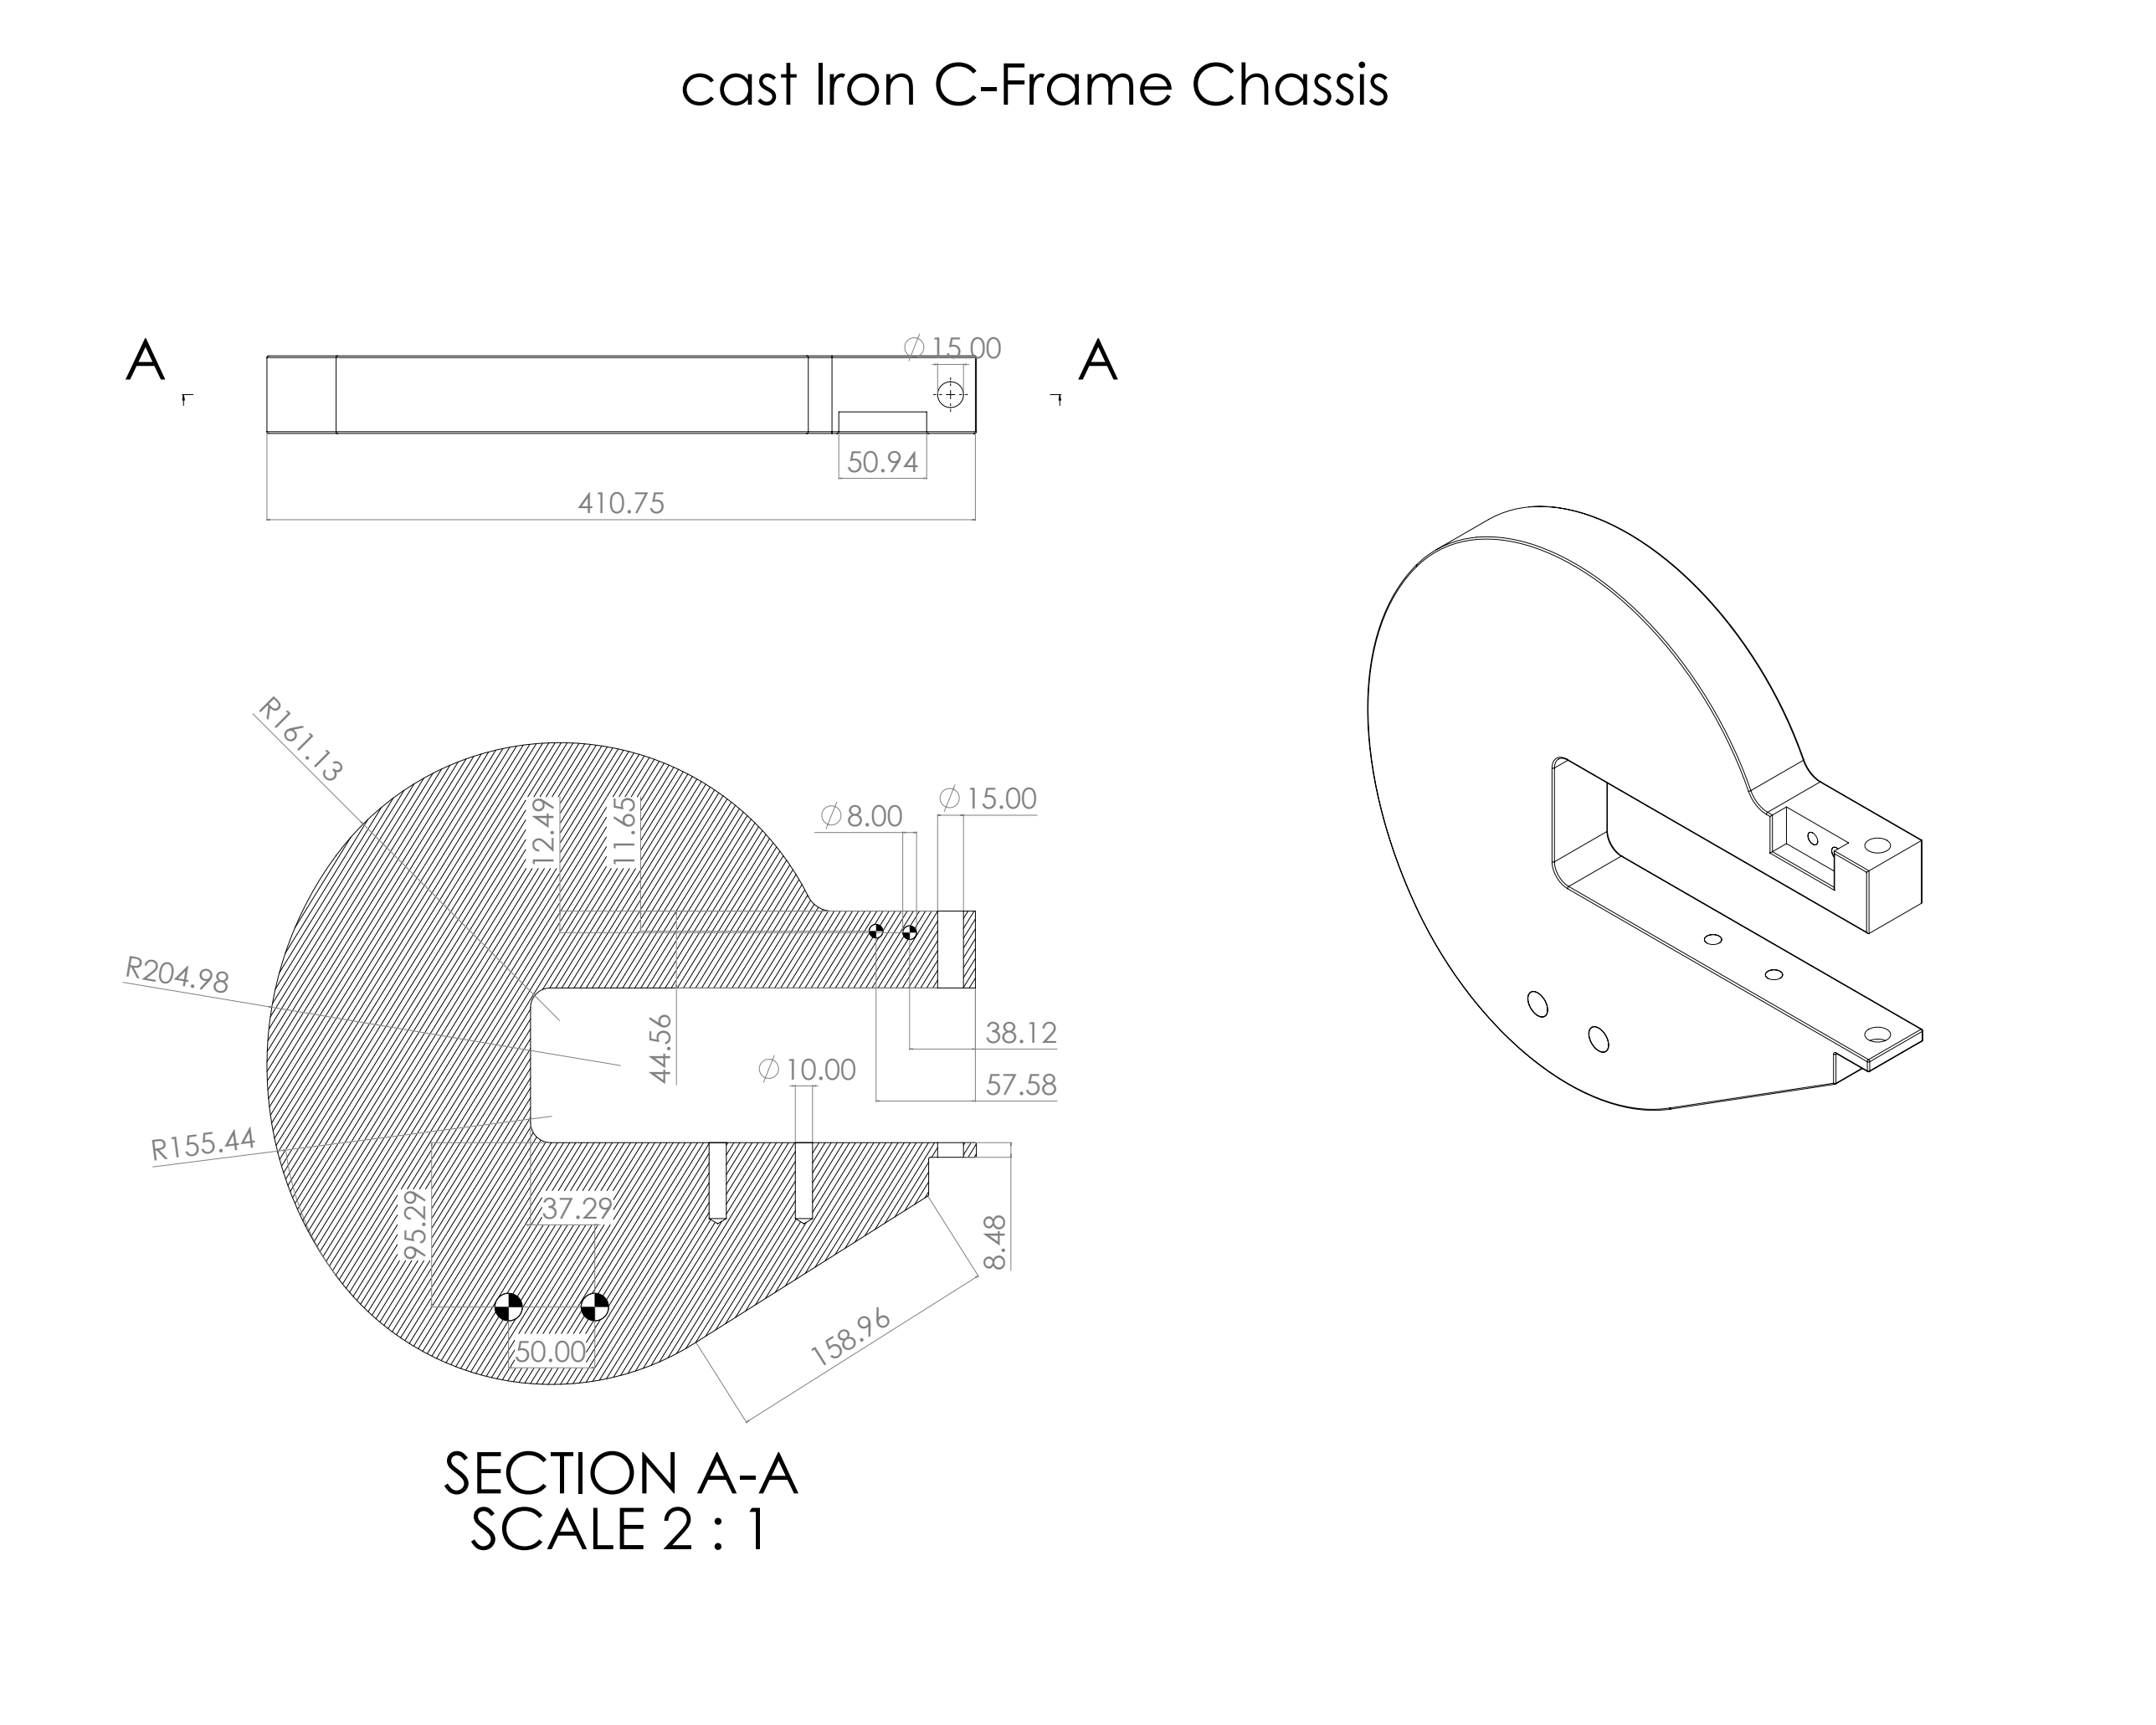
ISO-10303-21;
HEADER;
FILE_DESCRIPTION (('STEP AP214'),
    '1' );
FILE_NAME ('cast Iron C-Frame Chassis.step',
    '2026-10-25T20:52:49',
    ( '' ),
    ( '' ),
    'SwSTEP 2.0',
    'SolidWorks 2025',
    '' );
FILE_SCHEMA (( 'AUTOMOTIVE_DESIGN' ));
ENDSEC;

DATA;
#9=CARTESIAN_POINT ( 'NONE',  ( -147.0026986695708047, -210.7421749798627673, -22.50000000000000000 ) ) ;
#28=EDGE_CURVE ( 'NONE', #72058, #65497, #786, .T. ) ;
#32=DIRECTION ( 'NONE',  ( -0.8457827187922972723, -0.5335274993777825436, 0.000000000000000000 ) ) ;
#34=CARTESIAN_POINT ( 'NONE',  ( 143.2307367095235691, -26.41817448500847121, 22.50000000000000000 ) ) ;
#65=ADVANCED_FACE ( 'NONE', ( #14993 ), #6968, .F. ) ;
#67=CIRCLE ( 'NONE', #92305, 7.500000000000012434 ) ;
#69=ORIENTED_EDGE ( 'NONE', *, *, #59045, .F. ) ;
#114=PLANE ( 'NONE',  #30765 ) ;
#193=ORIENTED_EDGE ( 'NONE', *, *, #5103, .F. ) ;
#204=ORIENTED_EDGE ( 'NONE', *, *, #14407, .T. ) ;
#270=CIRCLE ( 'NONE', #69816, 1.000000000000001998 ) ;
#281=AXIS2_PLACEMENT_3D ( 'NONE', #4079, #26316, #18275 ) ;
#293=CARTESIAN_POINT ( 'NONE',  ( 169.2494399300530290, -11.64849832608277325, -3.999999999999998224 ) ) ;
#316=CARTESIAN_POINT ( 'NONE',  ( 139.6925840978351516, -0.9999999999999859002, -21.50000000000000000 ) ) ;
#333=AXIS2_PLACEMENT_3D ( 'NONE', #2350, #57785, #47737 ) ;
#361=ADVANCED_FACE ( 'NONE', ( #13917 ), #24780, .F. ) ;
#440=CIRCLE ( 'NONE', #73018, 5.024999999999987921 ) ;
#471=CYLINDRICAL_SURFACE ( 'NONE', #38369, 1.000000000000000888 ) ;
#500=CARTESIAN_POINT ( 'NONE',  ( 17.06571399127465583, -89.54582641780471874, -21.50000000000000000 ) ) ;
#501=VECTOR ( 'NONE', #78144, 1000.000000000000000 ) ;
#570=CIRCLE ( 'NONE', #62551, 4.025000000000000355 ) ;
#578=AXIS2_PLACEMENT_3D ( 'NONE', #28803, #50094, #12739 ) ;
#614=DIRECTION ( 'NONE',  ( 0.000000000000000000, 0.000000000000000000, 1.000000000000000000 ) ) ;
#651=ORIENTED_EDGE ( 'NONE', *, *, #66834, .T. ) ;
#770=( GEOMETRIC_REPRESENTATION_CONTEXT ( 3 ) GLOBAL_UNCERTAINTY_ASSIGNED_CONTEXT ( ( #62766 ) ) GLOBAL_UNIT_ASSIGNED_CONTEXT ( ( #61663, #3417, #24744 ) ) REPRESENTATION_CONTEXT ( 'NONE', 'WORKASPACE' ) );
#783=VERTEX_POINT ( 'NONE', #12506 ) ;
#786=CIRCLE ( 'NONE', #77907, 4.999999999999990230 ) ;
#792=CARTESIAN_POINT ( 'NONE',  ( 208.4306832106271088, 0.000000000000000000, 0.000000000000000000 ) ) ;
#799=EDGE_LOOP ( 'NONE', ( #93336, #90500 ) ) ;
#828=DIRECTION ( 'NONE',  ( 1.000000000000000000, -0.000000000000000000, -0.000000000000000000 ) ) ;
#853=ORIENTED_EDGE ( 'NONE', *, *, #21629, .T. ) ;
#914=EDGE_LOOP ( 'NONE', ( #28478, #27992, #72584 ) ) ;
#940=EDGE_CURVE ( 'NONE', #59842, #18158, #80294, .T. ) ;
#944=CARTESIAN_POINT ( 'NONE',  ( 195.7510731661265595, -142.7221692137691775, 21.50000000000000000 ) ) ;
#992=( BOUNDED_CURVE ( )  B_SPLINE_CURVE ( 3, ( #17869, #39604, #3665, #9823 ),
 .UNSPECIFIED., .F., .T. ) 
 B_SPLINE_CURVE_WITH_KNOTS ( ( 4, 4 ),
 ( 0.000000000000000000, 1.570796326794896558 ),
 .UNSPECIFIED. ) 
 CURVE ( )  GEOMETRIC_REPRESENTATION_ITEM ( )  RATIONAL_B_SPLINE_CURVE ( ( 1.000000000000000000, 0.8047378541243649375, 0.8047378541243649375, 1.000000000000000000 ) ) 
 REPRESENTATION_ITEM ( '' )  );
#993=ORIENTED_EDGE ( 'NONE', *, *, #1573, .T. ) ;
#996=( BOUNDED_CURVE ( )  B_SPLINE_CURVE ( 3, ( #21405, #22335, #16165, #31310 ),
 .UNSPECIFIED., .F., .F. ) 
 B_SPLINE_CURVE_WITH_KNOTS ( ( 4, 4 ),
 ( 1.570796326794896558, 3.141592653589793116 ),
 .UNSPECIFIED. ) 
 CURVE ( )  GEOMETRIC_REPRESENTATION_ITEM ( )  RATIONAL_B_SPLINE_CURVE ( ( 1.000000000000000000, 0.8047378541243649375, 0.8047378541243649375, 1.000000000000000000 ) ) 
 REPRESENTATION_ITEM ( '' )  );
#1053=CARTESIAN_POINT ( 'NONE',  ( 143.6449502718966755, 0.000000000000000000, 10.00000000000000178 ) ) ;
#1142=EDGE_CURVE ( 'NONE', #4350, #76692, #40467, .T. ) ;
#1221=VECTOR ( 'NONE', #34164, 1000.000000000000000 ) ;
#1245=CARTESIAN_POINT ( 'NONE',  ( -147.0026986695710320, 31.65052214425349675, 21.50000000000000000 ) ) ;
#1281=AXIS2_PLACEMENT_3D ( 'NONE', #34817, #63730, #27726 ) ;
#1304=FACE_BOUND ( 'NONE', #58441, .T. ) ;
#1348=VECTOR ( 'NONE', #50781, 1000.000000000000000 ) ;
#1363=DIRECTION ( 'NONE',  ( -0.000000000000000000, -1.000000000000000000, -0.000000000000000000 ) ) ;
#1389=DIRECTION ( 'NONE',  ( 0.000000000000000000, 0.000000000000000000, 1.000000000000000000 ) ) ;
#1391=CARTESIAN_POINT ( 'NONE',  ( 125.9462722777150958, 8.500086813760361792, 22.50000000000000000 ) ) ;
#1420=EDGE_CURVE ( 'NONE', #67590, #20083, #42046, .T. ) ;
#1458=DIRECTION ( 'NONE',  ( 0.000000000000000000, 1.000000000000000000, 0.000000000000000000 ) ) ;
#1463=ORIENTED_EDGE ( 'NONE', *, *, #63505, .T. ) ;
#1507=CARTESIAN_POINT ( 'NONE',  ( 228.6245981097501101, -142.7221692137691775, 21.50000000000000000 ) ) ;
#1573=EDGE_CURVE ( 'NONE', #90412, #43035, #24613, .T. ) ;
#1589=ORIENTED_EDGE ( 'NONE', *, *, #28, .T. ) ;
#1694=ORIENTED_EDGE ( 'NONE', *, *, #2190, .F. ) ;
#1706=ORIENTED_EDGE ( 'NONE', *, *, #90632, .F. ) ;
#1767=DIRECTION ( 'NONE',  ( 0.000000000000000000, 0.000000000000000000, 1.000000000000000000 ) ) ;
#1876=CIRCLE ( 'NONE', #32091, 1.000000000000000888 ) ;
#1918=EDGE_LOOP ( 'NONE', ( #64552, #5227, #88401, #55731 ) ) ;
#1948=AXIS2_PLACEMENT_3D ( 'NONE', #59364, #23828, #23372 ) ;
#1962=VECTOR ( 'NONE', #90749, 1000.000000000000000 ) ;
#1974=TOROIDAL_SURFACE ( 'NONE', #45753, 2.000000000000000000, 1.000000000000000000 ) ;
#2076=EDGE_CURVE ( 'NONE', #44526, #16441, #7114, .T. ) ;
#2081=CIRCLE ( 'NONE', #86680, 1.000000000000000888 ) ;
#2092=LINE ( 'NONE', #15363, #46809 ) ;
#2096=FACE_OUTER_BOUND ( 'NONE', #81756, .T. ) ;
#2171=LINE ( 'NONE', #86456, #14506 ) ;
#2175=EDGE_CURVE ( 'NONE', #55409, #59842, #55372, .T. ) ;
#2190=EDGE_CURVE ( 'NONE', #83649, #26494, #40004, .T. ) ;
#2228=EDGE_CURVE ( 'NONE', #26085, #32648, #28827, .T. ) ;
#2293=ADVANCED_FACE ( 'NONE', ( #78552 ), #42068, .F. ) ;
#2327=DIRECTION ( 'NONE',  ( -0.000000000000000000, -0.000000000000000000, 1.000000000000000000 ) ) ;
#2336=DIRECTION ( 'NONE',  ( 0.8429829950866641886, 0.5379402104274390028, -0.000000000000000000 ) ) ;
#2340=DIRECTION ( 'NONE',  ( -0.000000000000000000, 0.000000000000000000, 1.000000000000000000 ) ) ;
#2342=CARTESIAN_POINT ( 'NONE',  ( 208.4306832106271088, 0.000000000000000000, 0.000000000000000000 ) ) ;
#2350=CARTESIAN_POINT ( 'NONE',  ( 142.6449502718966755, 0.000000000000000000, 21.50000000000000000 ) ) ;
#2552=DIRECTION ( 'NONE',  ( -0.000000000000000000, -0.000000000000000000, 1.000000000000000000 ) ) ;
#2619=VERTEX_POINT ( 'NONE', #79936 ) ;
#2674=DIRECTION ( 'NONE',  ( -1.000000000000000000, -0.000000000000000000, -0.000000000000000000 ) ) ;
#2675=DIRECTION ( 'NONE',  ( -1.000000000000000000, 0.000000000000000000, 0.000000000000000000 ) ) ;
#2693=FACE_OUTER_BOUND ( 'NONE', #59104, .T. ) ;
#2706=EDGE_LOOP ( 'NONE', ( #8461, #84685, #42920, #69826 ) ) ;
#2712=EDGE_CURVE ( 'NONE', #71577, #17995, #44862, .T. ) ;
#2721=CARTESIAN_POINT ( 'NONE',  ( 194.5881128153457098, 0.000000000000000000, 10.00000000000000178 ) ) ;
#2846=ORIENTED_EDGE ( 'NONE', *, *, #39352, .F. ) ;
#2847=EDGE_CURVE ( 'NONE', #37463, #46977, #66092, .T. ) ;
#2871=FACE_OUTER_BOUND ( 'NONE', #72138, .T. ) ;
#3002=FACE_OUTER_BOUND ( 'NONE', #70187, .T. ) ;
#3092=AXIS2_PLACEMENT_3D ( 'NONE', #65272, #1767, #36359 ) ;
#3096=AXIS2_PLACEMENT_3D ( 'NONE', #75932, #24340, #53215 ) ;
#3148=CARTESIAN_POINT ( 'NONE',  ( 194.7510731661265595, -164.3527196417747405, 22.50000000000000000 ) ) ;
#3163=DIRECTION ( 'NONE',  ( 0.5335274993777934238, -0.8457827187922903889, 0.000000000000000000 ) ) ;
#3189=ORIENTED_EDGE ( 'NONE', *, *, #89909, .F. ) ;
#3220=CARTESIAN_POINT ( 'NONE',  ( -35.09237171215954731, -122.5496321078137356, 22.50000000000000000 ) ) ;
#3270=DIRECTION ( 'NONE',  ( -0.000000000000000000, -0.000000000000000000, -1.000000000000000000 ) ) ;
#3272=DIRECTION ( 'NONE',  ( 1.000000000000000000, 0.000000000000000000, 0.000000000000000000 ) ) ;
#3300=EDGE_LOOP ( 'NONE', ( #76937, #7294, #62037 ) ) ;
#3317=DIRECTION ( 'NONE',  ( 0.000000000000000000, 0.000000000000000000, 1.000000000000000000 ) ) ;
#3329=CARTESIAN_POINT ( 'NONE',  ( 222.4306832106270804, 15.36528803885690664, 21.50000000000000000 ) ) ;
#3355=AXIS2_PLACEMENT_3D ( 'NONE', #38183, #74661, #10239 ) ;
#3362=VECTOR ( 'NONE', #69642, 1000.000000000000000 ) ;
#3366=LINE ( 'NONE', #1507, #39639 ) ;
#3378=CARTESIAN_POINT ( 'NONE',  ( 60.83289261295102079, -250.0118895884541530, -21.50000000000000000 ) ) ;
#3393=DIRECTION ( 'NONE',  ( 0.000000000000000000, 0.000000000000000000, 1.000000000000000000 ) ) ;
#3417=( NAMED_UNIT ( * ) PLANE_ANGLE_UNIT ( ) SI_UNIT ( $, .RADIAN. ) );
#3430=AXIS2_PLACEMENT_3D ( 'NONE', #16645, #15259, #81046 ) ;
#3448=ORIENTED_EDGE ( 'NONE', *, *, #92749, .T. ) ;
#3465=( BOUNDED_CURVE ( )  B_SPLINE_CURVE ( 3, ( #12358, #18522, #40276, #48327 ),
 .UNSPECIFIED., .F., .F. ) 
 B_SPLINE_CURVE_WITH_KNOTS ( ( 4, 4 ),
 ( 1.570796326794896780, 3.141592653589793116 ),
 .UNSPECIFIED. ) 
 CURVE ( )  GEOMETRIC_REPRESENTATION_ITEM ( )  RATIONAL_B_SPLINE_CURVE ( ( 1.000000000000000000, 0.8047378541243650485, 0.8047378541243650485, 1.000000000000000000 ) ) 
 REPRESENTATION_ITEM ( '' )  );
#3479=CARTESIAN_POINT ( 'NONE',  ( 208.4306832106271088, 0.000000000000000000, 7.500000000000012434 ) ) ;
#3496=CONICAL_SURFACE ( 'NONE', #53370, 4.000000000000003553, 1.029744258676654534 ) ;
#3498=VERTEX_POINT ( 'NONE', #10746 ) ;
#3506=CARTESIAN_POINT ( 'NONE',  ( 139.6925840978351516, -0.9999999999999991118, 22.50000000000000000 ) ) ;
#3537=VERTEX_POINT ( 'NONE', #47665 ) ;
#3562=CONICAL_SURFACE ( 'NONE', #27780, 4.025000000000000355, 0.7853981633973095011 ) ;
#3569=DIRECTION ( 'NONE',  ( 0.000000000000000000, 0.000000000000000000, 1.000000000000000000 ) ) ;
#3635=EDGE_LOOP ( 'NONE', ( #75934, #12803, #4384, #93641 ) ) ;
#3665=CARTESIAN_POINT ( 'NONE',  ( 222.4201966301864672, -44.14345022962302068, 22.50000000000000000 ) ) ;
#3700=ORIENTED_EDGE ( 'NONE', *, *, #46910, .T. ) ;
#3716=SPHERICAL_SURFACE ( 'NONE', #83670, 1.000000000000000000 ) ;
#3802=DIRECTION ( 'NONE',  ( 1.000000000000000000, -1.124465274301078034E-16, -0.000000000000000000 ) ) ;
#3810=AXIS2_PLACEMENT_3D ( 'NONE', #50602, #62965, #14630 ) ;
#3858=CARTESIAN_POINT ( 'NONE',  ( -186.9122233887894140, -89.54582641780471874, 21.50000000000000000 ) ) ;
#3898=CYLINDRICAL_SURFACE ( 'NONE', #21924, 4.999999999999990230 ) ;
#3910=CARTESIAN_POINT ( 'NONE',  ( 123.4306832106270946, -178.2391364535880882, 0.000000000000000000 ) ) ;
#3923=DIRECTION ( 'NONE',  ( 1.000000000000000000, 0.000000000000000000, 0.000000000000000000 ) ) ;
#3948=CARTESIAN_POINT ( 'NONE',  ( 2.197429475817664013, -229.5268262511776527, 22.50000000000000000 ) ) ;
#3973=ORIENTED_EDGE ( 'NONE', *, *, #92308, .T. ) ;
#4015=EDGE_CURVE ( 'NONE', #20911, #3498, #27308, .T. ) ;
#4070=CARTESIAN_POINT ( 'NONE',  ( 10.19742947581766224, -229.5268262511776527, 22.47499999999998721 ) ) ;
#4079=CARTESIAN_POINT ( 'NONE',  ( 73.43068321062709458, -134.2391364535880598, 0.000000000000000000 ) ) ;
#4151=EDGE_CURVE ( 'NONE', #60845, #54318, #30836, .T. ) ;
#4179=FACE_BOUND ( 'NONE', #64618, .T. ) ;
#4193=FACE_OUTER_BOUND ( 'NONE', #12147, .T. ) ;
#4202=CARTESIAN_POINT ( 'NONE',  ( 223.4306832106270804, -141.7221692137691775, 21.50000000000000000 ) ) ;
#4227=LINE ( 'NONE', #33103, #24888 ) ;
#4306=CARTESIAN_POINT ( 'NONE',  ( -36.09237171215956863, -55.96374926131388605, 22.50000000000000000 ) ) ;
#4307=LINE ( 'NONE', #67779, #57934 ) ;
#4348=VERTEX_POINT ( 'NONE', #36269 ) ;
#4350=VERTEX_POINT ( 'NONE', #30561 ) ;
#4380=CARTESIAN_POINT ( 'NONE',  ( 222.8344101925596306, 0.000000000000000000, 21.50000000000000000 ) ) ;
#4384=ORIENTED_EDGE ( 'NONE', *, *, #60666, .F. ) ;
#4433=VERTEX_POINT ( 'NONE', #7388 ) ;
#4435=LINE ( 'NONE', #11542, #57938 ) ;
#4453=AXIS2_PLACEMENT_3D ( 'NONE', #13982, #86861, #13518 ) ;
#4493=ORIENTED_EDGE ( 'NONE', *, *, #8814, .T. ) ;
#4511=CIRCLE ( 'NONE', #30206, 1.000000000000000888 ) ;
#4532=EDGE_CURVE ( 'NONE', #63778, #79604, #52334, .T. ) ;
#4534=DIRECTION ( 'NONE',  ( 1.049727191138614998E-16, 0.5150380749100592626, -0.8571673007021092250 ) ) ;
#4562=ORIENTED_EDGE ( 'NONE', *, *, #31405, .F. ) ;
#4583=AXIS2_PLACEMENT_3D ( 'NONE', #12243, #84664, #56773 ) ;
#4592=ORIENTED_EDGE ( 'NONE', *, *, #28, .F. ) ;
#4661=CARTESIAN_POINT ( 'NONE',  ( 169.2494399300530290, -11.64849832608277325, 9.974999999999996092 ) ) ;
#4672=ORIENTED_EDGE ( 'NONE', *, *, #28909, .T. ) ;
#4716=EDGE_LOOP ( 'NONE', ( #87629, #16247, #76327, #79717 ) ) ;
#4734=DIRECTION ( 'NONE',  ( -0.000000000000000000, 1.000000000000000000, -0.000000000000000000 ) ) ;
#4800=CARTESIAN_POINT ( 'NONE',  ( -23.68628624284178130, -55.96374926131388605, -21.50000000000000000 ) ) ;
#4846=ORIENTED_EDGE ( 'NONE', *, *, #37797, .T. ) ;
#4847=CARTESIAN_POINT ( 'NONE',  ( 184.7149167944524493, -12.49482340714361506, -3.999999999999998224 ) ) ;
#4906=CARTESIAN_POINT ( 'NONE',  ( 139.6925840978351516, 15.36528803885690664, 21.50000000000000000 ) ) ;
#4922=CIRCLE ( 'NONE', #69947, 155.4364916446740210 ) ;
#4936=AXIS2_PLACEMENT_3D ( 'NONE', #87857, #44781, #58554 ) ;
#4941=EDGE_LOOP ( 'NONE', ( #13432, #18060, #5533, #32770 ) ) ;
#4964=VECTOR ( 'NONE', #8166, 1000.000000000000000 ) ;
#4982=AXIS2_PLACEMENT_3D ( 'NONE', #64437, #27960, #7553 ) ;
#5005=CARTESIAN_POINT ( 'NONE',  ( 223.4306832106270804, -134.2391364535880882, 21.50000000000000000 ) ) ;
#5053=ORIENTED_EDGE ( 'NONE', *, *, #31405, .T. ) ;
#5067=CIRCLE ( 'NONE', #41325, 5.024999999999987921 ) ;
#5068=DIRECTION ( 'NONE',  ( -0.000000000000000000, -0.000000000000000000, -1.000000000000000000 ) ) ;
#5089=VECTOR ( 'NONE', #77679, 1000.000000000000000 ) ;
#5090=EDGE_CURVE ( 'NONE', #63778, #72125, #60743, .T. ) ;
#5102=AXIS2_PLACEMENT_3D ( 'NONE', #7934, #51481, #30188 ) ;
#5103=EDGE_CURVE ( 'NONE', #85761, #66913, #89584, .T. ) ;
#5105=FACE_OUTER_BOUND ( 'NONE', #23551, .T. ) ;
#5135=DIRECTION ( 'NONE',  ( -0.000000000000000000, -0.000000000000000000, 1.000000000000000000 ) ) ;
#5177=CARTESIAN_POINT ( 'NONE',  ( 60.30377782462292657, -249.1633071459562530, -22.50000000000000000 ) ) ;
#5207=EDGE_CURVE ( 'NONE', #58726, #51305, #18800, .T. ) ;
#5214=EDGE_CURVE ( 'NONE', #77986, #22426, #29416, .T. ) ;
#5227=ORIENTED_EDGE ( 'NONE', *, *, #17969, .F. ) ;
#5231=VECTOR ( 'NONE', #32325, 1000.000000000000114 ) ;
#5245=VECTOR ( 'NONE', #31256, 1000.000000000000000 ) ;
#5278=FACE_OUTER_BOUND ( 'NONE', #81442, .T. ) ;
#5293=DIRECTION ( 'NONE',  ( -1.000000000000000000, 0.000000000000000000, 0.000000000000000000 ) ) ;
#5306=VECTOR ( 'NONE', #67620, 1000.000000000000000 ) ;
#5309=ORIENTED_EDGE ( 'NONE', *, *, #18425, .F. ) ;
#5345=EDGE_CURVE ( 'NONE', #87746, #70449, #23319, .T. ) ;
#5353=CARTESIAN_POINT ( 'NONE',  ( 194.5881128153457098, 0.000000000000000000, 21.50000000000000000 ) ) ;
#5415=DIRECTION ( 'NONE',  ( -0.000000000000000000, 1.000000000000000000, 0.000000000000000000 ) ) ;
#5433=VERTEX_POINT ( 'NONE', #85313 ) ;
#5455=ORIENTED_EDGE ( 'NONE', *, *, #35541, .T. ) ;
#5457=ADVANCED_FACE ( 'NONE', ( #55509 ), #65740, .F. ) ;
#5487=DIRECTION ( 'NONE',  ( -1.000000000000000000, 0.000000000000000000, 0.000000000000000000 ) ) ;
#5533=ORIENTED_EDGE ( 'NONE', *, *, #8883, .F. ) ;
#5558=ORIENTED_EDGE ( 'NONE', *, *, #18406, .T. ) ;
#5564=CARTESIAN_POINT ( 'NONE',  ( 200.9306832106270804, -324.2391364535881735, 0.000000000000000000 ) ) ;
#5591=DIRECTION ( 'NONE',  ( -1.000000000000000000, -1.187938636348916367E-11, 0.000000000000000000 ) ) ;
#5592=FACE_BOUND ( 'NONE', #39839, .T. ) ;
#5641=DIRECTION ( 'NONE',  ( -0.000000000000000000, -1.000000000000000000, -0.000000000000000000 ) ) ;
#5686=ORIENTED_EDGE ( 'NONE', *, *, #77753, .T. ) ;
#5687=ORIENTED_EDGE ( 'NONE', *, *, #23115, .T. ) ;
#5708=ADVANCED_FACE ( 'NONE', ( #56451 ), #26366, .T. ) ;
#5752=FACE_BOUND ( 'NONE', #81352, .T. ) ;
#5754=VECTOR ( 'NONE', #92574, 1000.000000000000000 ) ;
#5796=CARTESIAN_POINT ( 'NONE',  ( 222.4201966301864672, -0.4142135623730941463, 22.50000000000000000 ) ) ;
#5853=CARTESIAN_POINT ( 'NONE',  ( 222.8344101925596306, 0.000000000000000000, 22.50000000000000000 ) ) ;
#5915=VERTEX_POINT ( 'NONE', #42675 ) ;
#5949=DIRECTION ( 'NONE',  ( 0.000000000000000000, 0.000000000000000000, 1.000000000000000000 ) ) ;
#5960=DIRECTION ( 'NONE',  ( 0.000000000000000000, -0.000000000000000000, 1.000000000000000000 ) ) ;
#6016=ORIENTED_EDGE ( 'NONE', *, *, #53259, .F. ) ;
#6033=LINE ( 'NONE', #79407, #63830 ) ;
#6036=ORIENTED_EDGE ( 'NONE', *, *, #73376, .F. ) ;
#6037=LINE ( 'NONE', #56714, #26275 ) ;
#6092=FACE_OUTER_BOUND ( 'NONE', #24257, .T. ) ;
#6117=CYLINDRICAL_SURFACE ( 'NONE', #3810, 1.000000000000000888 ) ;
#6126=ORIENTED_EDGE ( 'NONE', *, *, #53259, .T. ) ;
#6151=VERTEX_POINT ( 'NONE', #51181 ) ;
#6218=DIRECTION ( 'NONE',  ( 1.000000000000000000, 0.000000000000000000, 0.000000000000000000 ) ) ;
#6271=DIRECTION ( 'NONE',  ( -1.000000000000000000, 0.000000000000000000, 0.000000000000000000 ) ) ;
#6292=AXIS2_PLACEMENT_3D ( 'NONE', #11680, #40530, #67591 ) ;
#6380=VERTEX_POINT ( 'NONE', #8098 ) ;
#6433=CIRCLE ( 'NONE', #56319, 1.000000000000000888 ) ;
#6488=VERTEX_POINT ( 'NONE', #51636 ) ;
#6489=CARTESIAN_POINT ( 'NONE',  ( 221.8344101925596306, -43.55766379199612004, -22.50000000000000000 ) ) ;
#6501=CIRCLE ( 'NONE', #18502, 7.500000000000012434 ) ;
#6503=EDGE_CURVE ( 'NONE', #67510, #7995, #59704, .T. ) ;
#6525=CIRCLE ( 'NONE', #50302, 1.000000000000000888 ) ;
#6564=AXIS2_PLACEMENT_3D ( 'NONE', #82409, #17556, #46408 ) ;
#6572=AXIS2_PLACEMENT_3D ( 'NONE', #54618, #75936, #26693 ) ;
#6578=DIRECTION ( 'NONE',  ( 0.000000000000000000, 0.000000000000000000, -1.000000000000000000 ) ) ;
#6592=DIRECTION ( 'NONE',  ( 0.000000000000000000, 0.000000000000000000, -1.000000000000000000 ) ) ;
#6600=AXIS2_PLACEMENT_3D ( 'NONE', #46808, #33548, #3272 ) ;
#6652=CIRCLE ( 'NONE', #82249, 0.9999999999999756861 ) ;
#6653=VECTOR ( 'NONE', #77496, 1000.000000000000000 ) ;
#6667=CARTESIAN_POINT ( 'NONE',  ( 222.4201966301864957, -0.4142135623730890392, -22.50000000000000000 ) ) ;
#6682=DIRECTION ( 'NONE',  ( -0.000000000000000000, 1.000000000000000000, -0.000000000000000000 ) ) ;
#6688=EDGE_CURVE ( 'NONE', #19742, #26019, #57841, .T. ) ;
#6707=AXIS2_PLACEMENT_3D ( 'NONE', #16995, #45861, #74768 ) ;
#6713=ORIENTED_EDGE ( 'NONE', *, *, #73275, .T. ) ;
#6752=CARTESIAN_POINT ( 'NONE',  ( 194.5881128153457098, -27.00396092263537540, 21.50000000000000000 ) ) ;
#6798=EDGE_CURVE ( 'NONE', #51305, #83756, #89011, .T. ) ;
#6827=ORIENTED_EDGE ( 'NONE', *, *, #19944, .T. ) ;
#6856=ORIENTED_EDGE ( 'NONE', *, *, #63349, .F. ) ;
#6869=EDGE_CURVE ( 'NONE', #27807, #55409, #9795, .T. ) ;
#6959=FACE_OUTER_BOUND ( 'NONE', #2706, .T. ) ;
#6968=CYLINDRICAL_SURFACE ( 'NONE', #21749, 7.999999999999992895 ) ;
#6970=ORIENTED_EDGE ( 'NONE', *, *, #15737, .F. ) ;
#7011=DIRECTION ( 'NONE',  ( -0.000000000000000000, -0.000000000000000000, -1.000000000000000000 ) ) ;
#7014=CARTESIAN_POINT ( 'NONE',  ( 215.9306832106271088, -134.2391364535880882, 9.184850993605173582E-16 ) ) ;
#7047=EDGE_CURVE ( 'NONE', #58642, #50388, #26025, .T. ) ;
#7084=( BOUNDED_CURVE ( )  B_SPLINE_CURVE ( 3, ( #71359, #70439, #28272, #6489 ),
 .UNSPECIFIED., .F., .F. ) 
 B_SPLINE_CURVE_WITH_KNOTS ( ( 4, 4 ),
 ( 0.000000000000000000, 1.570796326794896558 ),
 .UNSPECIFIED. ) 
 CURVE ( )  GEOMETRIC_REPRESENTATION_ITEM ( )  RATIONAL_B_SPLINE_CURVE ( ( 1.000000000000000000, 0.8047378541243649375, 0.8047378541243649375, 1.000000000000000000 ) ) 
 REPRESENTATION_ITEM ( '' )  );
#7088=ORIENTED_EDGE ( 'NONE', *, *, #81991, .T. ) ;
#7114=CIRCLE ( 'NONE', #19188, 161.1282194813176716 ) ;
#7154=EDGE_CURVE ( 'NONE', #70970, #15223, #24946, .T. ) ;
#7228=CARTESIAN_POINT ( 'NONE',  ( -35.09237171215954731, -55.96374926131388605, -21.49999999999998579 ) ) ;
#7274=EDGE_LOOP ( 'NONE', ( #29793, #86470, #92033, #65757 ) ) ;
#7277=ORIENTED_EDGE ( 'NONE', *, *, #28588, .T. ) ;
#7294=ORIENTED_EDGE ( 'NONE', *, *, #45328, .T. ) ;
#7336=CARTESIAN_POINT ( 'NONE',  ( 17.06571399127465583, -89.54582641780471874, -21.50000000000000000 ) ) ;
#7388=CARTESIAN_POINT ( 'NONE',  ( 221.8344101925596306, -0.9999999999999997780, -22.50000000000000000 ) ) ;
#7404=DIRECTION ( 'NONE',  ( -1.000000000000000000, 0.000000000000000000, 0.000000000000000000 ) ) ;
#7418=EDGE_LOOP ( 'NONE', ( #20822, #91078, #16702, #11786 ) ) ;
#7436=FACE_BOUND ( 'NONE', #16047, .T. ) ;
#7451=CARTESIAN_POINT ( 'NONE',  ( 161.2244399300530233, -11.64849832608277325, 10.00000000000000000 ) ) ;
#7473=ORIENTED_EDGE ( 'NONE', *, *, #55430, .F. ) ;
#7522=DIRECTION ( 'NONE',  ( -0.000000000000000000, -0.000000000000000000, -1.000000000000000000 ) ) ;
#7536=ORIENTED_EDGE ( 'NONE', *, *, #57188, .T. ) ;
#7553=DIRECTION ( 'NONE',  ( 0.000000000000000000, 0.000000000000000000, -1.000000000000000000 ) ) ;
#7564=AXIS2_PLACEMENT_3D ( 'NONE', #75251, #90812, #46350 ) ;
#7612=( BOUNDED_CURVE ( )  B_SPLINE_CURVE ( 3, ( #81407, #52998, #81872, #44499 ),
 .UNSPECIFIED., .F., .F. ) 
 B_SPLINE_CURVE_WITH_KNOTS ( ( 4, 4 ),
 ( 4.712388980384689674, 6.283185307179586232 ),
 .UNSPECIFIED. ) 
 CURVE ( )  GEOMETRIC_REPRESENTATION_ITEM ( )  RATIONAL_B_SPLINE_CURVE ( ( 1.000000000000000000, 0.8047378541243649375, 0.8047378541243649375, 1.000000000000000000 ) ) 
 REPRESENTATION_ITEM ( '' )  );
#7625=AXIS2_PLACEMENT_3D ( 'NONE', #91159, #85489, #5960 ) ;
#7692=ORIENTED_EDGE ( 'NONE', *, *, #26979, .F. ) ;
#7694=AXIS2_PLACEMENT_3D ( 'NONE', #31819, #17148, #54054 ) ;
#7767=AXIS2_PLACEMENT_3D ( 'NONE', #76083, #25875, #75155 ) ;
#7776=CARTESIAN_POINT ( 'NONE',  ( -6.024775384615294271, -229.5268262511776527, 22.50000000000000000 ) ) ;
#7934=CARTESIAN_POINT ( 'NONE',  ( 196.7510731661265595, -143.7221692137691775, -22.50000000000000000 ) ) ;
#7994=ORIENTED_EDGE ( 'NONE', *, *, #24610, .F. ) ;
#7995=VERTEX_POINT ( 'NONE', #4202 ) ;
#8021=AXIS2_PLACEMENT_3D ( 'NONE', #42595, #86150, #50174 ) ;
#8023=CARTESIAN_POINT ( 'NONE',  ( 222.4306832106270804, -135.2391364535880882, 22.50000000000000000 ) ) ;
#8048=EDGE_CURVE ( 'NONE', #60407, #70970, #74830, .T. ) ;
#8064=VERTEX_POINT ( 'NONE', #68138 ) ;
#8091=EDGE_LOOP ( 'NONE', ( #18639, #18013, #41578, #5687 ) ) ;
#8098=CARTESIAN_POINT ( 'NONE',  ( 143.6449502718966755, 0.000000000000000000, 10.00000000000000178 ) ) ;
#8123=FACE_OUTER_BOUND ( 'NONE', #12515, .T. ) ;
#8166=DIRECTION ( 'NONE',  ( -0.7071067811864494290, 8.659560562353731078E-17, 0.7071067811866457165 ) ) ;
#8202=ORIENTED_EDGE ( 'NONE', *, *, #79416, .F. ) ;
#8235=ORIENTED_EDGE ( 'NONE', *, *, #69736, .T. ) ;
#8249=DIRECTION ( 'NONE',  ( -1.000000000000000000, 0.000000000000000000, 0.000000000000000000 ) ) ;
#8264=DIRECTION ( 'NONE',  ( -0.000000000000000000, -0.000000000000000000, -1.000000000000000000 ) ) ;
#8461=ORIENTED_EDGE ( 'NONE', *, *, #84910, .T. ) ;
#8477=DIRECTION ( 'NONE',  ( 1.000000000000000000, 0.000000000000000000, 0.000000000000000000 ) ) ;
#8540=ORIENTED_EDGE ( 'NONE', *, *, #48693, .T. ) ;
#8592=CYLINDRICAL_SURFACE ( 'NONE', #83655, 1.000000000000000888 ) ;
#8616=FACE_OUTER_BOUND ( 'NONE', #22304, .T. ) ;
#8700=EDGE_CURVE ( 'NONE', #32853, #8064, #59421, .T. ) ;
#8709=DIRECTION ( 'NONE',  ( -0.000000000000000000, -0.000000000000000000, 1.000000000000000000 ) ) ;
#8730=CYLINDRICAL_SURFACE ( 'NONE', #13741, 1.000000000000000888 ) ;
#8814=EDGE_CURVE ( 'NONE', #10408, #37463, #89190, .T. ) ;
#8822=DIRECTION ( 'NONE',  ( -0.000000000000000000, -0.000000000000000000, -1.000000000000000000 ) ) ;
#8883=EDGE_CURVE ( 'NONE', #4350, #82047, #24343, .T. ) ;
#8902=AXIS2_PLACEMENT_3D ( 'NONE', #60794, #17703, #46556 ) ;
#8903=DIRECTION ( 'NONE',  ( 0.000000000000000000, 1.000000000000000000, 0.000000000000000000 ) ) ;
#8911=CYLINDRICAL_SURFACE ( 'NONE', #66977, 1.000000000000000888 ) ;
#8931=DIRECTION ( 'NONE',  ( 0.4467993836324665735, -0.8946341770721976117, 0.000000000000000000 ) ) ;
#8964=AXIS2_PLACEMENT_3D ( 'NONE', #59774, #74900, #31800 ) ;
#8988=CARTESIAN_POINT ( 'NONE',  ( 194.7510731661265595, -164.3527196417747689, 21.50000000000000000 ) ) ;
#9057=LINE ( 'NONE', #73023, #89652 ) ;
#9067=LINE ( 'NONE', #37945, #46744 ) ;
#9090=AXIS2_PLACEMENT_3D ( 'NONE', #25554, #91818, #55862 ) ;
#9137=ORIENTED_EDGE ( 'NONE', *, *, #28588, .F. ) ;
#9149=LINE ( 'NONE', #24784, #83506 ) ;
#9164=AXIS2_PLACEMENT_3D ( 'NONE', #51355, #93513, #79342 ) ;
#9205=EDGE_CURVE ( 'NONE', #90412, #75708, #23881, .T. ) ;
#9240=ORIENTED_EDGE ( 'NONE', *, *, #15737, .T. ) ;
#9252=CARTESIAN_POINT ( 'NONE',  ( 73.43068321062708037, -181.2434395487258598, 0.000000000000000000 ) ) ;
#9328=VERTEX_POINT ( 'NONE', #3506 ) ;
#9433=AXIS2_PLACEMENT_3D ( 'NONE', #66174, #52406, #37719 ) ;
#9448=LINE ( 'NONE', #9925, #5245 ) ;
#9453=DIRECTION ( 'NONE',  ( 0.000000000000000000, 0.000000000000000000, 1.000000000000000000 ) ) ;
#9500=AXIS2_PLACEMENT_3D ( 'NONE', #35832, #92640, #73570 ) ;
#9511=AXIS2_PLACEMENT_3D ( 'NONE', #18831, #24049, #74242 ) ;
#9513=DIRECTION ( 'NONE',  ( 0.000000000000000000, -1.000000000000000000, 0.000000000000000000 ) ) ;
#9541=DIRECTION ( 'NONE',  ( -0.000000000000000000, 1.000000000000000000, -0.000000000000000000 ) ) ;
#9555=AXIS2_PLACEMENT_3D ( 'NONE', #82064, #56365, #74989 ) ;
#9557=DIRECTION ( 'NONE',  ( -0.000000000000000000, -0.000000000000000000, -1.000000000000000000 ) ) ;
#9558=DIRECTION ( 'NONE',  ( -1.000000000000000000, 0.000000000000000000, 0.000000000000000000 ) ) ;
#9581=AXIS2_PLACEMENT_3D ( 'NONE', #23741, #25139, #16177 ) ;
#9602=EDGE_LOOP ( 'NONE', ( #32888, #36068, #7692, #53755 ) ) ;
#9635=ADVANCED_FACE ( 'NONE', ( #54160 ), #77348, .T. ) ;
#9644=EDGE_CURVE ( 'NONE', #16441, #2619, #86634, .T. ) ;
#9702=VERTEX_POINT ( 'NONE', #18183 ) ;
#9720=AXIS2_PLACEMENT_3D ( 'NONE', #11752, #47248, #40605 ) ;
#9744=DIRECTION ( 'NONE',  ( -1.000000000000000000, 0.000000000000000000, 0.000000000000000000 ) ) ;
#9753=DIRECTION ( 'NONE',  ( 0.000000000000000000, 0.000000000000000000, 1.000000000000000000 ) ) ;
#9782=DIRECTION ( 'NONE',  ( -0.000000000000000000, -0.000000000000000000, 1.000000000000000000 ) ) ;
#9785=DIRECTION ( 'NONE',  ( 0.000000000000000000, 0.000000000000000000, 1.000000000000000000 ) ) ;
#9795=CIRCLE ( 'NONE', #29490, 4.999999999999990230 ) ;
#9823=CARTESIAN_POINT ( 'NONE',  ( 221.8344101925596306, -43.55766379199612004, 22.50000000000000000 ) ) ;
#9853=DIRECTION ( 'NONE',  ( 0.000000000000000000, -1.000000000000000000, 0.000000000000000000 ) ) ;
#9884=EDGE_CURVE ( 'NONE', #43035, #26246, #4435, .T. ) ;
#9888=LINE ( 'NONE', #74285, #68682 ) ;
#9925=CARTESIAN_POINT ( 'NONE',  ( 223.4306832106270804, -147.4436952405746979, 21.50000000000000000 ) ) ;
#9966=LINE ( 'NONE', #80535, #23168 ) ;
#9975=DIRECTION ( 'NONE',  ( 0.000000000000000000, 0.000000000000000000, 1.000000000000000000 ) ) ;
#10058=ORIENTED_EDGE ( 'NONE', *, *, #70761, .T. ) ;
#10110=CARTESIAN_POINT ( 'NONE',  ( 194.7510731661265595, -164.3527196417747689, -22.50000000000000000 ) ) ;
#10130=CARTESIAN_POINT ( 'NONE',  ( 123.4306832106270946, -134.2391364535880882, 0.000000000000000000 ) ) ;
#10164=ORIENTED_EDGE ( 'NONE', *, *, #49321, .F. ) ;
#10219=DIRECTION ( 'NONE',  ( -0.000000000000000000, -0.000000000000000000, 1.000000000000000000 ) ) ;
#10239=DIRECTION ( 'NONE',  ( 0.000000000000000000, 0.000000000000000000, 1.000000000000000000 ) ) ;
#10266=EDGE_LOOP ( 'NONE', ( #14633, #78886, #92170, #83436 ) ) ;
#10339=DIRECTION ( 'NONE',  ( -0.000000000000000000, -0.000000000000000000, -1.000000000000000000 ) ) ;
#10365=ORIENTED_EDGE ( 'NONE', *, *, #40665, .F. ) ;
#10366=DIRECTION ( 'NONE',  ( -1.000000000000000000, 0.000000000000000000, 0.000000000000000000 ) ) ;
#10381=CARTESIAN_POINT ( 'NONE',  ( 222.4306832106270804, -135.2391364535880882, -21.50000000000000000 ) ) ;
#10384=ADVANCED_FACE ( 'NONE', ( #60446 ), #71600, .T. ) ;
#10389=DIRECTION ( 'NONE',  ( -0.5335274993777934238, 0.8457827187922903889, 0.000000000000000000 ) ) ;
#10408=VERTEX_POINT ( 'NONE', #87885 ) ;
#10427=DIRECTION ( 'NONE',  ( 0.000000000000000000, 0.000000000000000000, 1.000000000000000000 ) ) ;
#10535=EDGE_CURVE ( 'NONE', #76692, #61220, #51887, .T. ) ;
#10556=DIRECTION ( 'NONE',  ( 0.000000000000000000, 0.000000000000000000, -1.000000000000000000 ) ) ;
#10594=CARTESIAN_POINT ( 'NONE',  ( 123.4306832106270946, -178.2391364535880882, -4.999999999999990230 ) ) ;
#10596=ORIENTED_EDGE ( 'NONE', *, *, #73376, .T. ) ;
#10693=DIRECTION ( 'NONE',  ( -1.000000000000000000, 0.000000000000000000, 0.000000000000000000 ) ) ;
#10696=DIRECTION ( 'NONE',  ( 0.000000000000000000, 1.000000000000000000, 0.000000000000000000 ) ) ;
#10707=EDGE_CURVE ( 'NONE', #15284, #27807, #90669, .T. ) ;
#10746=CARTESIAN_POINT ( 'NONE',  ( 73.43068321062709458, -178.2391364535880882, -4.999999999999990230 ) ) ;
#10796=FACE_OUTER_BOUND ( 'NONE', #914, .T. ) ;
#10819=LINE ( 'NONE', #17941, #18494 ) ;
#10822=DIRECTION ( 'NONE',  ( -0.000000000000000000, -0.000000000000000000, -1.000000000000000000 ) ) ;
#10971=ORIENTED_EDGE ( 'NONE', *, *, #90632, .T. ) ;
#10982=AXIS2_PLACEMENT_3D ( 'NONE', #57536, #14456, #43313 ) ;
#11023=AXIS2_PLACEMENT_3D ( 'NONE', #8988, #11797, #10389 ) ;
#11034=DIRECTION ( 'NONE',  ( -0.000000000000000000, -0.000000000000000000, -1.000000000000000000 ) ) ;
#11042=DIRECTION ( 'NONE',  ( 1.000000000000000000, 0.000000000000000000, 0.000000000000000000 ) ) ;
#11056=AXIS2_PLACEMENT_3D ( 'NONE', #16292, #45145, #60326 ) ;
#11057=ORIENTED_EDGE ( 'NONE', *, *, #32100, .F. ) ;
#11078=CIRCLE ( 'NONE', #57949, 1.000000000000000888 ) ;
#11096=CIRCLE ( 'NONE', #6600, 4.000000000000003553 ) ;
#11098=ORIENTED_EDGE ( 'NONE', *, *, #84781, .T. ) ;
#11165=CARTESIAN_POINT ( 'NONE',  ( -22.78264641048746597, -118.9815703160634541, 22.50000000000000000 ) ) ;
#11241=AXIS2_PLACEMENT_3D ( 'NONE', #77241, #62588, #91431 ) ;
#11280=CARTESIAN_POINT ( 'NONE',  ( -147.0026986695707762, 31.65052214425332622, -22.50000000000000000 ) ) ;
#11361=AXIS2_PLACEMENT_3D ( 'NONE', #57143, #5068, #85984 ) ;
#11424=PLANE ( 'NONE',  #65478 ) ;
#11438=CARTESIAN_POINT ( 'NONE',  ( 139.6925840978351516, -0.9999999999999991118, 21.50000000000000000 ) ) ;
#11454=ORIENTED_EDGE ( 'NONE', *, *, #89540, .F. ) ;
#11506=AXIS2_PLACEMENT_3D ( 'NONE', #48238, #84693, #79014 ) ;
#11542=CARTESIAN_POINT ( 'NONE',  ( 194.7510731661265595, 15.36528803885690664, 22.50000000000000000 ) ) ;
#11577=EDGE_CURVE ( 'NONE', #40890, #70302, #44390, .T. ) ;
#11646=FACE_BOUND ( 'NONE', #799, .T. ) ;
#11668=DIRECTION ( 'NONE',  ( -1.000000000000000000, 0.000000000000000000, 0.000000000000000000 ) ) ;
#11680=CARTESIAN_POINT ( 'NONE',  ( 222.4306832106270804, -135.2391364535880882, 22.50000000000000000 ) ) ;
#11718=CARTESIAN_POINT ( 'NONE',  ( 195.7510731661265595, -141.7221692137691775, -22.50000000000000000 ) ) ;
#11752=CARTESIAN_POINT ( 'NONE',  ( -22.78264641048746597, -118.9815703160634541, -22.50000000000000000 ) ) ;
#11786=ORIENTED_EDGE ( 'NONE', *, *, #16494, .F. ) ;
#11797=DIRECTION ( 'NONE',  ( -0.8457827187922973833, -0.5335274993777826547, -0.000000000000000000 ) ) ;
#11814=PRODUCT_CONTEXT ( 'NONE', #58995, 'mechanical' ) ;
#11818=VECTOR ( 'NONE', #27744, 999.9999999999998863 ) ;
#11835=CARTESIAN_POINT ( 'NONE',  ( 73.43068321062709458, -134.2391364535880598, 0.000000000000000000 ) ) ;
#11883=CIRCLE ( 'NONE', #88986, 8.222204860432944074 ) ;
#11942=ORIENTED_EDGE ( 'NONE', *, *, #22600, .T. ) ;
#11950=CARTESIAN_POINT ( 'NONE',  ( 223.4306832106270804, -141.7221692137691775, -21.50000000000000000 ) ) ;
#11984=ORIENTED_EDGE ( 'NONE', *, *, #67622, .F. ) ;
#12024=CARTESIAN_POINT ( 'NONE',  ( 194.7510731661265595, -143.7221692137691775, -21.50000000000000000 ) ) ;
#12106=CARTESIAN_POINT ( 'NONE',  ( 123.4306832106270946, -178.2391364535880882, -4.999999999999990230 ) ) ;
#12147=EDGE_LOOP ( 'NONE', ( #10058, #18795, #73951, #70782 ) ) ;
#12192=ORIENTED_EDGE ( 'NONE', *, *, #34350, .F. ) ;
#12243=CARTESIAN_POINT ( 'NONE',  ( -23.68628624284178130, -55.96374926131388605, -21.50000000000000000 ) ) ;
#12262=EDGE_CURVE ( 'NONE', #9702, #46866, #996, .T. ) ;
#12282=PRODUCT_DEFINITION ( 'UNKNOWN', '', #55311, #56106 ) ;
#12358=CARTESIAN_POINT ( 'NONE',  ( 142.6449502718966755, -0.9999999999999991118, 22.50000000000000000 ) ) ;
#12373=LINE ( 'NONE', #70158, #1221 ) ;
#12399=ORIENTED_EDGE ( 'NONE', *, *, #51127, .T. ) ;
#12434=CIRCLE ( 'NONE', #17020, 1.000000000000000888 ) ;
#12438=DIRECTION ( 'NONE',  ( -1.000000000000000000, 0.000000000000000000, 0.000000000000000000 ) ) ;
#12442=ADVANCED_FACE ( 'NONE', ( #73480 ), #8592, .T. ) ;
#12499=VECTOR ( 'NONE', #23598, 1000.000000000000000 ) ;
#12504=CIRCLE ( 'NONE', #65458, 0.9999999999999896749 ) ;
#12506=CARTESIAN_POINT ( 'NONE',  ( 180.7149167944524493, -12.49482340714361506, 9.974999999999996092 ) ) ;
#12515=EDGE_LOOP ( 'NONE', ( #47451, #72161, #50155, #89688 ) ) ;
#12558=VECTOR ( 'NONE', #2327, 1000.000000000000000 ) ;
#12663=ORIENTED_EDGE ( 'NONE', *, *, #61955, .T. ) ;
#12671=AXIS2_PLACEMENT_3D ( 'NONE', #12024, #5415, #62226 ) ;
#12686=EDGE_CURVE ( 'NONE', #44672, #9702, #66378, .T. ) ;
#12739=DIRECTION ( 'NONE',  ( -1.000000000000000000, 0.000000000000000000, 0.000000000000000000 ) ) ;
#12748=AXIS2_PLACEMENT_3D ( 'NONE', #65973, #86780, #19704 ) ;
#12803=ORIENTED_EDGE ( 'NONE', *, *, #37560, .F. ) ;
#12827=AXIS2_PLACEMENT_3D ( 'NONE', #33571, #79493, #86098 ) ;
#12856=CARTESIAN_POINT ( 'NONE',  ( -186.9122233887894140, -89.54582641780471874, -21.50000000000000000 ) ) ;
#12891=CLOSED_SHELL ( 'NONE', ( #10384, #55547, #52294, #52932, #69157, #65, #91315, #23330, #5457, #87661, #20887, #25465, #65910, #36404, #88027, #50712, #73319, #74739, #15971, #51544, #56439, #20906, #78512, #62357, #38799, #26815, #84374, #51967, #23454, #44619, #24725, #66306, #82902, #76916, #71878, #71024, #78352, #77875, #50999, #93461, #93687, #65131, #36314, #57046, #85549, #48216, #36009, #53886, #73628, #56259, #72074, #87370, #2293, #361, #39249, #82139, #29537, #78861, #44512, #45415, #32468, #66676, #60125, #59950, #64549, #31870, #61165, #88420, #61089, #64336, #85860, #19859, #58095, #83200, #9635, #13313, #70090, #80042, #61953, #48034, #71460, #20269, #25549, #12442, #93296, #53587, #25147, #61188, #44387, #89731, #39023, #77158, #62925, #5708, #60651, #80248, #61339, #12996, #23035, #32868, #60761, #78811, #15814, #43232, #48494, #42514, #85563, #41728, #88796 ) ) ;
#12908=VERTEX_POINT ( 'NONE', #41173 ) ;
#12942=EDGE_CURVE ( 'NONE', #25794, #79714, #33168, .T. ) ;
#12952=DIRECTION ( 'NONE',  ( 0.000000000000000000, 1.000000000000000000, 0.000000000000000000 ) ) ;
#12996=ADVANCED_FACE ( 'NONE', ( #91856 ), #63494, .T. ) ;
#13142=DIRECTION ( 'NONE',  ( 1.000000000000000000, 0.000000000000000000, 0.000000000000000000 ) ) ;
#13150=LINE ( 'NONE', #92183, #19924 ) ;
#13169=DIRECTION ( 'NONE',  ( -0.8457827187922973833, -0.5335274993777826547, 0.000000000000000000 ) ) ;
#13282=CARTESIAN_POINT ( 'NONE',  ( 222.8344101925596306, -44.55766379199612004, 21.50000000000000000 ) ) ;
#13291=LINE ( 'NONE', #28426, #41404 ) ;
#13313=ADVANCED_FACE ( 'NONE', ( #92325 ), #471, .T. ) ;
#13331=EDGE_CURVE ( 'NONE', #3498, #55409, #13291, .T. ) ;
#13385=DIRECTION ( 'NONE',  ( -0.000000000000000000, -0.000000000000000000, -1.000000000000000000 ) ) ;
#13403=CARTESIAN_POINT ( 'NONE',  ( -56.02477538461528184, -229.5268262511776527, 22.50000000000000000 ) ) ;
#13432=ORIENTED_EDGE ( 'NONE', *, *, #12942, .T. ) ;
#13434=VERTEX_POINT ( 'NONE', #8023 ) ;
#13448=CARTESIAN_POINT ( 'NONE',  ( -47.80257052418233599, -229.5268262511776527, 21.50000000000000000 ) ) ;
#13518=DIRECTION ( 'NONE',  ( 0.000000000000000000, 0.000000000000000000, 1.000000000000000000 ) ) ;
#13531=CIRCLE ( 'NONE', #37686, 4.025000000000000355 ) ;
#13579=FACE_OUTER_BOUND ( 'NONE', #9602, .T. ) ;
#13627=CARTESIAN_POINT ( 'NONE',  ( 60.30156426812556703, -249.1647034777049328, -21.50000000000000000 ) ) ;
#13651=DIRECTION ( 'NONE',  ( 0.5941640067486205767, 0.8043439146810431595, 0.000000000000000000 ) ) ;
#13668=FACE_OUTER_BOUND ( 'NONE', #74197, .T. ) ;
#13725=ORIENTED_EDGE ( 'NONE', *, *, #14175, .T. ) ;
#13741=AXIS2_PLACEMENT_3D ( 'NONE', #80245, #79787, #14477 ) ;
#13747=CARTESIAN_POINT ( 'NONE',  ( 194.7510731661265595, -143.7221692137691775, -22.50000000000000000 ) ) ;
#13759=DIRECTION ( 'NONE',  ( -1.000000000000000000, 0.000000000000000000, 0.000000000000000000 ) ) ;
#13794=CARTESIAN_POINT ( 'NONE',  ( 222.4306832106270804, -135.2391364535880882, 21.50000000000000000 ) ) ;
#13866=CIRCLE ( 'NONE', #66772, 1.000000000000000888 ) ;
#13874=DIRECTION ( 'NONE',  ( -0.000000000000000000, -0.000000000000000000, -1.000000000000000000 ) ) ;
#13917=FACE_OUTER_BOUND ( 'NONE', #47419, .T. ) ;
#13927=ORIENTED_EDGE ( 'NONE', *, *, #35541, .F. ) ;
#13982=CARTESIAN_POINT ( 'NONE',  ( 73.43068321062709458, -178.2391364535880882, 0.000000000000000000 ) ) ;
#13993=EDGE_CURVE ( 'NONE', #90518, #43675, #64190, .T. ) ;
#13999=CIRCLE ( 'NONE', #75954, 0.9999999999999980016 ) ;
#14056=ORIENTED_EDGE ( 'NONE', *, *, #92749, .F. ) ;
#14079=DIRECTION ( 'NONE',  ( -0.000000000000000000, -1.000000000000000000, -0.000000000000000000 ) ) ;
#14140=CARTESIAN_POINT ( 'NONE',  ( 139.6925840978351516, -0.9999999999999991118, 22.50000000000000000 ) ) ;
#14167=AXIS2_PLACEMENT_3D ( 'NONE', #29712, #74650, #38650 ) ;
#14175=EDGE_CURVE ( 'NONE', #90412, #22436, #59633, .T. ) ;
#14235=DIRECTION ( 'NONE',  ( 1.124465274301078034E-16, 1.000000000000000000, 0.000000000000000000 ) ) ;
#14274=DIRECTION ( 'NONE',  ( 0.000000000000000000, 0.5150380749100522682, 0.8571673007021134438 ) ) ;
#14365=ORIENTED_EDGE ( 'NONE', *, *, #75740, .T. ) ;
#14374=AXIS2_PLACEMENT_3D ( 'NONE', #35915, #57701, #42533 ) ;
#14387=CARTESIAN_POINT ( 'NONE',  ( 184.7149167944524493, -12.49482340714361506, 10.00000000000000000 ) ) ;
#14407=EDGE_CURVE ( 'NONE', #57485, #87117, #76237, .T. ) ;
#14431=VERTEX_POINT ( 'NONE', #23162 ) ;
#14434=ORIENTED_EDGE ( 'NONE', *, *, #13331, .F. ) ;
#14456=DIRECTION ( 'NONE',  ( 0.000000000000000000, 0.000000000000000000, 1.000000000000000000 ) ) ;
#14477=DIRECTION ( 'NONE',  ( 0.000000000000000000, 0.000000000000000000, -1.000000000000000000 ) ) ;
#14506=VECTOR ( 'NONE', #22539, 1000.000000000000000 ) ;
#14534=DIRECTION ( 'NONE',  ( -1.000000000000000000, 0.000000000000000000, 0.000000000000000000 ) ) ;
#14630=DIRECTION ( 'NONE',  ( 0.000000000000000000, -1.000000000000000000, 0.000000000000000000 ) ) ;
#14633=ORIENTED_EDGE ( 'NONE', *, *, #27345, .F. ) ;
#14648=EDGE_CURVE ( 'NONE', #83649, #16441, #62679, .T. ) ;
#14651=VERTEX_POINT ( 'NONE', #18873 ) ;
#14652=LINE ( 'NONE', #43508, #60503 ) ;
#14666=ORIENTED_EDGE ( 'NONE', *, *, #51127, .F. ) ;
#14824=CYLINDRICAL_SURFACE ( 'NONE', #24617, 1.000000000000000888 ) ;
#14876=ORIENTED_EDGE ( 'NONE', *, *, #69834, .T. ) ;
#14899=DIRECTION ( 'NONE',  ( -0.000000000000000000, -0.000000000000000000, -1.000000000000000000 ) ) ;
#14909=EDGE_CURVE ( 'NONE', #57485, #37428, #50557, .T. ) ;
#14910=DIRECTION ( 'NONE',  ( -0.000000000000000000, -0.000000000000000000, -1.000000000000000000 ) ) ;
#14983=DIRECTION ( 'NONE',  ( 1.000000000000000000, 0.000000000000000000, 0.000000000000000000 ) ) ;
#14993=FACE_OUTER_BOUND ( 'NONE', #59363, .T. ) ;
#15076=AXIS2_PLACEMENT_3D ( 'NONE', #70242, #12952, #28542 ) ;
#15111=VERTEX_POINT ( 'NONE', #91750 ) ;
#15163=EDGE_CURVE ( 'NONE', #70449, #60290, #91272, .T. ) ;
#15182=LINE ( 'NONE', #85739, #89891 ) ;
#15223=VERTEX_POINT ( 'NONE', #17932 ) ;
#15259=DIRECTION ( 'NONE',  ( 0.000000000000000000, -1.000000000000000000, 0.000000000000000000 ) ) ;
#15270=CYLINDRICAL_SURFACE ( 'NONE', #8964, 4.999999999999990230 ) ;
#15284=VERTEX_POINT ( 'NONE', #78960 ) ;
#15309=ORIENTED_EDGE ( 'NONE', *, *, #77753, .F. ) ;
#15337=ORIENTED_EDGE ( 'NONE', *, *, #79978, .T. ) ;
#15363=CARTESIAN_POINT ( 'NONE',  ( 139.6925840978351516, -27.00396092263537184, 22.50000000000000000 ) ) ;
#15484=LINE ( 'NONE', #30623, #92521 ) ;
#15519=ORIENTED_EDGE ( 'NONE', *, *, #30767, .F. ) ;
#15533=AXIS2_PLACEMENT_3D ( 'NONE', #15559, #73336, #8903 ) ;
#15559=CARTESIAN_POINT ( 'NONE',  ( 223.4306832106270804, -135.2391364535880882, -21.50000000000000000 ) ) ;
#15737=EDGE_CURVE ( 'NONE', #46977, #81769, #87975, .T. ) ;
#15740=ORIENTED_EDGE ( 'NONE', *, *, #37853, .T. ) ;
#15742=DIRECTION ( 'NONE',  ( 0.000000000000000000, 1.000000000000000000, 0.000000000000000000 ) ) ;
#15763=DIRECTION ( 'NONE',  ( -0.000000000000000000, -0.000000000000000000, 1.000000000000000000 ) ) ;
#15775=CIRCLE ( 'NONE', #59658, 4.999999999999990230 ) ;
#15814=ADVANCED_FACE ( 'NONE', ( #79441 ), #78883, .T. ) ;
#15832=VECTOR ( 'NONE', #3802, 1000.000000000000000 ) ;
#15843=CIRCLE ( 'NONE', #68758, 4.025000000000000355 ) ;
#15865=CARTESIAN_POINT ( 'NONE',  ( 139.6925840978351516, -43.55766379199612004, 22.50000000000000000 ) ) ;
#15954=DIRECTION ( 'NONE',  ( -0.000000000000000000, -1.000000000000000000, -0.000000000000000000 ) ) ;
#15971=ADVANCED_FACE ( 'NONE', ( #59524 ), #23523, .F. ) ;
#15990=CARTESIAN_POINT ( 'NONE',  ( 125.0516381006429043, 8.053287430127898716, 22.50000000000000000 ) ) ;
#16015=ORIENTED_EDGE ( 'NONE', *, *, #5207, .F. ) ;
#16017=EDGE_CURVE ( 'NONE', #65497, #41863, #15484, .T. ) ;
#16047=EDGE_LOOP ( 'NONE', ( #11098, #86357 ) ) ;
#16070=CARTESIAN_POINT ( 'NONE',  ( -147.0026986695710320, 31.65052214425349675, 22.50000000000000000 ) ) ;
#16165=CARTESIAN_POINT ( 'NONE',  ( 194.5881128153456814, -26.00396092263537895, 22.08578643762690419 ) ) ;
#16177=DIRECTION ( 'NONE',  ( -1.000000000000000000, 0.000000000000000000, 0.000000000000000000 ) ) ;
#16188=CARTESIAN_POINT ( 'NONE',  ( 143.6449502718966755, -26.00396092263537540, 21.50000000000000000 ) ) ;
#16205=CARTESIAN_POINT ( 'NONE',  ( 223.4306832106270804, -141.7221692137691775, 22.50000000000000000 ) ) ;
#16247=ORIENTED_EDGE ( 'NONE', *, *, #15163, .F. ) ;
#16292=CARTESIAN_POINT ( 'NONE',  ( 17.06571399127465583, -89.54582641780471874, -21.50000000000000000 ) ) ;
#16295=DIRECTION ( 'NONE',  ( -1.000000000000000000, 0.000000000000000000, 0.000000000000000000 ) ) ;
#16349=ORIENTED_EDGE ( 'NONE', *, *, #87626, .F. ) ;
#16385=ORIENTED_EDGE ( 'NONE', *, *, #44575, .F. ) ;
#16441=VERTEX_POINT ( 'NONE', #52851 ) ;
#16494=EDGE_CURVE ( 'NONE', #44867, #75656, #74170, .T. ) ;
#16518=CARTESIAN_POINT ( 'NONE',  ( 169.2494399300530290, -11.64849832608277325, 10.00000000000000000 ) ) ;
#16538=FACE_OUTER_BOUND ( 'NONE', #79504, .T. ) ;
#16557=CIRCLE ( 'NONE', #51353, 4.999999999999990230 ) ;
#16616=AXIS2_PLACEMENT_3D ( 'NONE', #60693, #6682, #70610 ) ;
#16633=CYLINDRICAL_SURFACE ( 'NONE', #9581, 7.500000000000007105 ) ;
#16645=CARTESIAN_POINT ( 'NONE',  ( -6.024775384615294271, -229.5268262511776527, 21.50000000000000000 ) ) ;
#16655=DIRECTION ( 'NONE',  ( 0.000000000000000000, 0.000000000000000000, 1.000000000000000000 ) ) ;
#16658=DIRECTION ( 'NONE',  ( 0.000000000000000000, 0.000000000000000000, -1.000000000000000000 ) ) ;
#16691=EDGE_LOOP ( 'NONE', ( #38062, #78353, #27341, #48439 ) ) ;
#16696=EDGE_CURVE ( 'NONE', #7995, #73033, #74335, .T. ) ;
#16702=ORIENTED_EDGE ( 'NONE', *, *, #63505, .F. ) ;
#16744=DIRECTION ( 'NONE',  ( 1.000000000000000000, 0.000000000000000000, 0.000000000000000000 ) ) ;
#16754=AXIS2_PLACEMENT_3D ( 'NONE', #10130, #59890, #83025 ) ;
#16793=EDGE_CURVE ( 'NONE', #82488, #77986, #33410, .T. ) ;
#16809=EDGE_LOOP ( 'NONE', ( #41523, #65504, #55717, #80992 ) ) ;
#16811=ORIENTED_EDGE ( 'NONE', *, *, #41200, .T. ) ;
#16816=EDGE_CURVE ( 'NONE', #18158, #59842, #42574, .T. ) ;
#16889=CARTESIAN_POINT ( 'NONE',  ( -147.8070425842520308, 32.24468615100210656, -21.49999999999998579 ) ) ;
#16892=CYLINDRICAL_SURFACE ( 'NONE', #3355, 1.000000000000000888 ) ;
#16930=DIRECTION ( 'NONE',  ( 0.000000000000000000, -0.000000000000000000, -1.000000000000000000 ) ) ;
#16966=ORIENTED_EDGE ( 'NONE', *, *, #38034, .T. ) ;
#16967=FACE_OUTER_BOUND ( 'NONE', #31728, .T. ) ;
#16995=CARTESIAN_POINT ( 'NONE',  ( 61.37083282337847123, -250.8548725835408391, -22.50000000000000000 ) ) ;
#17018=ORIENTED_EDGE ( 'NONE', *, *, #20108, .F. ) ;
#17020=AXIS2_PLACEMENT_3D ( 'NONE', #45280, #46225, #9785 ) ;
#17027=VECTOR ( 'NONE', #15954, 1000.000000000000000 ) ;
#17035=ORIENTED_EDGE ( 'NONE', *, *, #85914, .T. ) ;
#17086=TOROIDAL_SURFACE ( 'NONE', #11056, 203.9779373800640485, 1.000000000000000000 ) ;
#17095=VECTOR ( 'NONE', #45170, 1000.000000000000114 ) ;
#17132=LINE ( 'NONE', #16205, #92672 ) ;
#17148=DIRECTION ( 'NONE',  ( -0.000000000000000000, -0.000000000000000000, -1.000000000000000000 ) ) ;
#17225=DIRECTION ( 'NONE',  ( -0.000000000000000000, -0.000000000000000000, -1.000000000000000000 ) ) ;
#17244=CIRCLE ( 'NONE', #91290, 7.500000000000012434 ) ;
#17263=CIRCLE ( 'NONE', #80781, 11.40608546931776779 ) ;
#17324=DIRECTION ( 'NONE',  ( 1.000000000000000000, 0.000000000000000000, 0.000000000000000000 ) ) ;
#17370=DIRECTION ( 'NONE',  ( 0.000000000000000000, 1.000000000000000000, 0.000000000000000000 ) ) ;
#17373=DIRECTION ( 'NONE',  ( 0.000000000000000000, 0.000000000000000000, 1.000000000000000000 ) ) ;
#17471=DIRECTION ( 'NONE',  ( -0.5379402104274362273, 0.8429829950866658539, 0.000000000000000000 ) ) ;
#17500=CYLINDRICAL_SURFACE ( 'NONE', #24682, 7.999999999999992895 ) ;
#17529=EDGE_LOOP ( 'NONE', ( #53252, #29553 ) ) ;
#17539=ORIENTED_EDGE ( 'NONE', *, *, #20409, .T. ) ;
#17556=DIRECTION ( 'NONE',  ( -1.000000000000000000, 0.000000000000000000, 0.000000000000000000 ) ) ;
#17644=DIRECTION ( 'NONE',  ( 0.000000000000000000, 0.000000000000000000, 1.000000000000000000 ) ) ;
#17655=CARTESIAN_POINT ( 'NONE',  ( 180.7149167944524493, -12.49482340714361506, -3.999999999999998224 ) ) ;
#17703=DIRECTION ( 'NONE',  ( 0.000000000000000000, 0.000000000000000000, 1.000000000000000000 ) ) ;
#17738=DIRECTION ( 'NONE',  ( -1.000000000000000000, 0.000000000000000000, 0.000000000000000000 ) ) ;
#17817=CARTESIAN_POINT ( 'NONE',  ( 194.7510731661265595, -143.7221692137691775, 21.50000000000000000 ) ) ;
#17843=AXIS2_PLACEMENT_3D ( 'NONE', #39353, #68271, #3393 ) ;
#17869=CARTESIAN_POINT ( 'NONE',  ( 222.8344101925596306, -44.55766379199612004, 21.50000000000000000 ) ) ;
#17887=LINE ( 'NONE', #83198, #5306 ) ;
#17932=CARTESIAN_POINT ( 'NONE',  ( 125.0516381006427338, 8.053287430127817004, -22.50000000000000000 ) ) ;
#17941=CARTESIAN_POINT ( 'NONE',  ( -187.9122233887894140, -89.54582641780471874, 22.50000000000000000 ) ) ;
#17969=EDGE_CURVE ( 'NONE', #73033, #20083, #3366, .T. ) ;
#17976=CARTESIAN_POINT ( 'NONE',  ( -18.20453976106250948, -63.49190233628851132, 21.50000000000000000 ) ) ;
#17995=VERTEX_POINT ( 'NONE', #16188 ) ;
#17996=EDGE_LOOP ( 'NONE', ( #14365, #88855, #13927, #21694 ) ) ;
#17997=CARTESIAN_POINT ( 'NONE',  ( 222.8344101925596306, 0.000000000000000000, 21.50000000000000000 ) ) ;
#18013=ORIENTED_EDGE ( 'NONE', *, *, #54005, .T. ) ;
#18060=ORIENTED_EDGE ( 'NONE', *, *, #23274, .T. ) ;
#18098=CARTESIAN_POINT ( 'NONE',  ( 73.43068321062709458, -178.2391364535880882, 0.000000000000000000 ) ) ;
#18101=AXIS2_PLACEMENT_3D ( 'NONE', #500, #67234, #44951 ) ;
#18124=ORIENTED_EDGE ( 'NONE', *, *, #47455, .F. ) ;
#18125=FACE_OUTER_BOUND ( 'NONE', #93299, .T. ) ;
#18140=DIRECTION ( 'NONE',  ( -0.000000000000000000, -0.000000000000000000, -1.000000000000000000 ) ) ;
#18158=VERTEX_POINT ( 'NONE', #39325 ) ;
#18183=CARTESIAN_POINT ( 'NONE',  ( 195.5881128153457098, -27.00396092263537540, 22.50000000000000000 ) ) ;
#18275=DIRECTION ( 'NONE',  ( 0.000000000000000000, 0.000000000000000000, 1.000000000000000000 ) ) ;
#18301=VERTEX_POINT ( 'NONE', #4306 ) ;
#18376=DIRECTION ( 'NONE',  ( 1.000000000000000000, 0.000000000000000000, 0.000000000000000000 ) ) ;
#18392=CARTESIAN_POINT ( 'NONE',  ( -47.80257052418233599, -229.5268262511776527, -22.50000000000000000 ) ) ;
#18406=EDGE_CURVE ( 'NONE', #48629, #83166, #44192, .T. ) ;
#18425=EDGE_CURVE ( 'NONE', #44526, #43675, #70598, .T. ) ;
#18494=VECTOR ( 'NONE', #68602, 1000.000000000000000 ) ;
#18502=AXIS2_PLACEMENT_3D ( 'NONE', #792, #21160, #51419 ) ;
#18522=CARTESIAN_POINT ( 'NONE',  ( 143.2307367095235406, -0.4142135623730943128, 22.50000000000000000 ) ) ;
#18533=SPHERICAL_SURFACE ( 'NONE', #53551, 1.000000000000000000 ) ;
#18534=EDGE_CURVE ( 'NONE', #25794, #32648, #6433, .T. ) ;
#18557=CARTESIAN_POINT ( 'NONE',  ( -187.9122233887894140, -89.54582641780471874, 21.50000000000000000 ) ) ;
#18579=CIRCLE ( 'NONE', #63976, 8.222204860432958284 ) ;
#18590=VERTEX_POINT ( 'NONE', #92338 ) ;
#18609=AXIS2_PLACEMENT_3D ( 'NONE', #54978, #34149, #69656 ) ;
#18635=AXIS2_PLACEMENT_3D ( 'NONE', #38279, #8931, #37809 ) ;
#18639=ORIENTED_EDGE ( 'NONE', *, *, #76268, .T. ) ;
#18664=DIRECTION ( 'NONE',  ( 0.000000000000000000, -1.000000000000000000, 0.000000000000000000 ) ) ;
#18722=CIRCLE ( 'NONE', #83730, 4.000000000000003553 ) ;
#18763=LINE ( 'NONE', #55220, #11818 ) ;
#18795=ORIENTED_EDGE ( 'NONE', *, *, #68972, .F. ) ;
#18800=CIRCLE ( 'NONE', #70256, 1.000000000000000888 ) ;
#18808=AXIS2_PLACEMENT_3D ( 'NONE', #18963, #61589, #63480 ) ;
#18821=CIRCLE ( 'NONE', #12748, 8.222204860432958284 ) ;
#18831=CARTESIAN_POINT ( 'NONE',  ( -47.80257052418233599, -229.5268262511776527, 22.47499999999998721 ) ) ;
#18839=LINE ( 'NONE', #84608, #74473 ) ;
#18844=DIRECTION ( 'NONE',  ( -0.000000000000000000, -0.000000000000000000, 1.000000000000000000 ) ) ;
#18873=CARTESIAN_POINT ( 'NONE',  ( 195.7510731661265595, -164.3527196417747405, -21.50000000000000000 ) ) ;
#18875=CARTESIAN_POINT ( 'NONE',  ( 184.7149167944524493, -12.49482340714361506, 9.974999999999996092 ) ) ;
#18910=DIRECTION ( 'NONE',  ( -1.000000000000000000, 0.000000000000000000, 0.000000000000000000 ) ) ;
#18940=AXIS2_PLACEMENT_3D ( 'NONE', #90959, #40773, #33703 ) ;
#18942=DIRECTION ( 'NONE',  ( -0.000000000000000000, -0.000000000000000000, -1.000000000000000000 ) ) ;
#18963=CARTESIAN_POINT ( 'NONE',  ( 2.197429475817664013, -229.5268262511776527, 22.47499999999998721 ) ) ;
#19006=DIRECTION ( 'NONE',  ( -1.000000000000000000, 0.000000000000000000, 0.000000000000000000 ) ) ;
#19045=ORIENTED_EDGE ( 'NONE', *, *, #7154, .F. ) ;
#19095=FACE_OUTER_BOUND ( 'NONE', #21021, .T. ) ;
#19120=ORIENTED_EDGE ( 'NONE', *, *, #84897, .T. ) ;
#19188=AXIS2_PLACEMENT_3D ( 'NONE', #17976, #54415, #55837 ) ;
#19244=ORIENTED_EDGE ( 'NONE', *, *, #27513, .F. ) ;
#19314=DIRECTION ( 'NONE',  ( 0.000000000000000000, 0.000000000000000000, 1.000000000000000000 ) ) ;
#19327=DIRECTION ( 'NONE',  ( 0.000000000000000000, 0.000000000000000000, 1.000000000000000000 ) ) ;
#19347=ORIENTED_EDGE ( 'NONE', *, *, #60229, .T. ) ;
#19413=FACE_OUTER_BOUND ( 'NONE', #84459, .T. ) ;
#19422=CARTESIAN_POINT ( 'NONE',  ( 222.4306832106270804, -135.2391364535880882, -21.50000000000000000 ) ) ;
#19448=CARTESIAN_POINT ( 'NONE',  ( -147.8070425842520308, 32.24468615100210656, 22.50000000000000000 ) ) ;
#19512=ORIENTED_EDGE ( 'NONE', *, *, #38034, .F. ) ;
#19524=ORIENTED_EDGE ( 'NONE', *, *, #55430, .T. ) ;
#19558=CARTESIAN_POINT ( 'NONE',  ( 194.5881128153457098, -26.00396092263537540, -47.19625681453479871 ) ) ;
#19574=FACE_OUTER_BOUND ( 'NONE', #37045, .T. ) ;
#19593=DIRECTION ( 'NONE',  ( -1.000000000000000000, 0.000000000000000000, 0.000000000000000000 ) ) ;
#19637=ORIENTED_EDGE ( 'NONE', *, *, #84489, .F. ) ;
#19683=LINE ( 'NONE', #42386, #5754 ) ;
#19704=DIRECTION ( 'NONE',  ( -1.000000000000000000, 0.000000000000000000, 0.000000000000000000 ) ) ;
#19742=VERTEX_POINT ( 'NONE', #33977 ) ;
#19763=DIRECTION ( 'NONE',  ( -1.000000000000000000, 0.000000000000000000, 0.000000000000000000 ) ) ;
#19791=EDGE_CURVE ( 'NONE', #81769, #68679, #18579, .T. ) ;
#19812=EDGE_CURVE ( 'NONE', #89567, #46866, #18839, .T. ) ;
#19859=ADVANCED_FACE ( 'NONE', ( #34904 ), #20075, .T. ) ;
#19886=DIRECTION ( 'NONE',  ( 0.000000000000000000, 0.000000000000000000, -1.000000000000000000 ) ) ;
#19908=EDGE_CURVE ( 'NONE', #6488, #5433, #49573, .T. ) ;
#19924=VECTOR ( 'NONE', #78469, 1000.000000000000000 ) ;
#19925=EDGE_LOOP ( 'NONE', ( #47310, #79631, #38502, #77134 ) ) ;
#19926=CARTESIAN_POINT ( 'NONE',  ( 60.83509176750334291, -250.0104861964972258, 22.50000000000000000 ) ) ;
#19929=CARTESIAN_POINT ( 'NONE',  ( 61.37083282337847123, -250.8548725835408391, 21.50000000000000000 ) ) ;
#19932=VECTOR ( 'NONE', #4534, 999.9999999999998863 ) ;
#19941=DIRECTION ( 'NONE',  ( -0.000000000000000000, -1.000000000000000000, -0.000000000000000000 ) ) ;
#19944=EDGE_CURVE ( 'NONE', #37793, #58642, #24591, .T. ) ;
#19999=AXIS2_PLACEMENT_3D ( 'NONE', #20747, #57216, #49618 ) ;
#20004=CARTESIAN_POINT ( 'NONE',  ( 215.9306832106271088, -142.7221692137691775, 9.184850993605173582E-16 ) ) ;
#20017=DIRECTION ( 'NONE',  ( 0.000000000000000000, -1.000000000000000000, 0.000000000000000000 ) ) ;
#20023=DIRECTION ( 'NONE',  ( -0.8457827187922972723, -0.5335274993777825436, -0.000000000000000000 ) ) ;
#20040=ORIENTED_EDGE ( 'NONE', *, *, #79416, .T. ) ;
#20075=TOROIDAL_SURFACE ( 'NONE', #88109, 203.9779373800640485, 1.000000000000000000 ) ;
#20080=ORIENTED_EDGE ( 'NONE', *, *, #8048, .T. ) ;
#20083=VERTEX_POINT ( 'NONE', #50967 ) ;
#20108=EDGE_CURVE ( 'NONE', #3537, #46977, #43397, .T. ) ;
#20138=DIRECTION ( 'NONE',  ( 0.000000000000000000, 0.000000000000000000, 1.000000000000000000 ) ) ;
#20192=ORIENTED_EDGE ( 'NONE', *, *, #76386, .T. ) ;
#20202=AXIS2_PLACEMENT_3D ( 'NONE', #23635, #2336, #17471 ) ;
#20269=ADVANCED_FACE ( 'NONE', ( #36757 ), #80551, .T. ) ;
#20271=EDGE_CURVE ( 'NONE', #29017, #74706, #6501, .T. ) ;
#20274=CARTESIAN_POINT ( 'NONE',  ( 194.5881128153457098, 0.000000000000000000, 10.00000000000000178 ) ) ;
#20294=AXIS2_PLACEMENT_3D ( 'NONE', #83714, #26903, #69995 ) ;
#20381=VECTOR ( 'NONE', #30789, 1000.000000000000000 ) ;
#20409=EDGE_CURVE ( 'NONE', #75708, #83756, #76029, .T. ) ;
#20415=CARTESIAN_POINT ( 'NONE',  ( 142.6449502718966755, -27.00396092263537540, 22.50000000000000000 ) ) ;
#20695=DIRECTION ( 'NONE',  ( 0.000000000000000000, 0.000000000000000000, -1.000000000000000000 ) ) ;
#20696=CARTESIAN_POINT ( 'NONE',  ( 222.8344101925596306, 0.000000000000000000, 21.50000000000000000 ) ) ;
#20736=DIRECTION ( 'NONE',  ( -0.000000000000000000, -0.000000000000000000, -1.000000000000000000 ) ) ;
#20747=CARTESIAN_POINT ( 'NONE',  ( 228.6245981097501101, -142.7221692137691775, -32.50000000000000711 ) ) ;
#20785=CARTESIAN_POINT ( 'NONE',  ( 223.4306832106270804, -135.2391364535880882, 22.50000000000000000 ) ) ;
#20822=ORIENTED_EDGE ( 'NONE', *, *, #81991, .F. ) ;
#20885=DIRECTION ( 'NONE',  ( -0.000000000000000000, -0.000000000000000000, 1.000000000000000000 ) ) ;
#20887=ADVANCED_FACE ( 'NONE', ( #59954 ), #68437, .F. ) ;
#20900=ORIENTED_EDGE ( 'NONE', *, *, #79581, .T. ) ;
#20906=ADVANCED_FACE ( 'NONE', ( #81693 ), #89721, .F. ) ;
#20911=VERTEX_POINT ( 'NONE', #9252 ) ;
#20964=LINE ( 'NONE', #78728, #36226 ) ;
#21021=EDGE_LOOP ( 'NONE', ( #11984, #48862, #42087 ) ) ;
#21160=DIRECTION ( 'NONE',  ( 0.000000000000000000, -1.000000000000000000, 0.000000000000000000 ) ) ;
#21164=ORIENTED_EDGE ( 'NONE', *, *, #34074, .T. ) ;
#21195=DIRECTION ( 'NONE',  ( 1.000000000000000000, 0.000000000000000000, 0.000000000000000000 ) ) ;
#21222=FACE_OUTER_BOUND ( 'NONE', #73438, .T. ) ;
#21224=DIRECTION ( 'NONE',  ( -0.000000000000000000, -0.000000000000000000, -1.000000000000000000 ) ) ;
#21234=VERTEX_POINT ( 'NONE', #63710 ) ;
#21258=EDGE_LOOP ( 'NONE', ( #52221, #92460, #86091, #65744 ) ) ;
#21267=ORIENTED_EDGE ( 'NONE', *, *, #54642, .T. ) ;
#21373=EDGE_LOOP ( 'NONE', ( #41245, #41609, #90007, #91075 ) ) ;
#21379=CARTESIAN_POINT ( 'NONE',  ( 2.197429475817664013, -229.5268262511776527, 21.50000000000000000 ) ) ;
#21391=ORIENTED_EDGE ( 'NONE', *, *, #11577, .F. ) ;
#21405=CARTESIAN_POINT ( 'NONE',  ( 195.5881128153457098, -27.00396092263537540, 22.50000000000000000 ) ) ;
#21447=CARTESIAN_POINT ( 'NONE',  ( 180.6899167944524436, -12.49482340714361506, 10.00000000000000000 ) ) ;
#21458=EDGE_LOOP ( 'NONE', ( #83410, #80515, #49232, #24152 ) ) ;
#21629=EDGE_CURVE ( 'NONE', #18301, #32853, #92567, .T. ) ;
#21694=ORIENTED_EDGE ( 'NONE', *, *, #85093, .F. ) ;
#21749=AXIS2_PLACEMENT_3D ( 'NONE', #57625, #86468, #65682 ) ;
#21789=VECTOR ( 'NONE', #30275, 1000.000000000000000 ) ;
#21845=VECTOR ( 'NONE', #28775, 1000.000000000000000 ) ;
#21875=AXIS2_PLACEMENT_3D ( 'NONE', #78090, #49657, #93211 ) ;
#21907=LINE ( 'NONE', #28544, #30080 ) ;
#21924=AXIS2_PLACEMENT_3D ( 'NONE', #54537, #82496, #31843 ) ;
#21929=VECTOR ( 'NONE', #92173, 1000.000000000000000 ) ;
#21960=ORIENTED_EDGE ( 'NONE', *, *, #54119, .F. ) ;
#22006=CARTESIAN_POINT ( 'NONE',  ( 73.43068321062709458, -178.2391364535880882, 0.000000000000000000 ) ) ;
#22075=DIRECTION ( 'NONE',  ( 0.8571673007021122226, 0.000000000000000000, 0.5150380749100541555 ) ) ;
#22101=DIRECTION ( 'NONE',  ( -0.000000000000000000, 1.000000000000000000, -0.000000000000000000 ) ) ;
#22118=DIRECTION ( 'NONE',  ( -0.000000000000000000, 0.000000000000000000, -1.000000000000000000 ) ) ;
#22134=FACE_OUTER_BOUND ( 'NONE', #27505, .T. ) ;
#22169=ORIENTED_EDGE ( 'NONE', *, *, #54639, .T. ) ;
#22170=CARTESIAN_POINT ( 'NONE',  ( 188.7399167944524550, -12.49482340714361506, 10.00000000000000000 ) ) ;
#22232=CARTESIAN_POINT ( 'NONE',  ( 161.2494399300530290, -11.64849832608277325, 9.974999999999996092 ) ) ;
#22285=DIRECTION ( 'NONE',  ( 0.000000000000000000, 0.000000000000000000, -1.000000000000000000 ) ) ;
#22304=EDGE_LOOP ( 'NONE', ( #47280, #28968, #11942, #31716 ) ) ;
#22333=CYLINDRICAL_SURFACE ( 'NONE', #32391, 1.000000000000000888 ) ;
#22335=CARTESIAN_POINT ( 'NONE',  ( 195.0023263777187879, -26.41817448500847121, 22.50000000000000000 ) ) ;
#22354=CARTESIAN_POINT ( 'NONE',  ( 17.06571399127465583, -89.54582641780471874, -22.50000000000000000 ) ) ;
#22374=EDGE_CURVE ( 'NONE', #14651, #75846, #1876, .T. ) ;
#22426=VERTEX_POINT ( 'NONE', #74982 ) ;
#22436=VERTEX_POINT ( 'NONE', #66936 ) ;
#22475=EDGE_CURVE ( 'NONE', #78431, #59355, #9149, .T. ) ;
#22481=CARTESIAN_POINT ( 'NONE',  ( 139.6925840978351516, -0.9999999999999859002, -22.50000000000000000 ) ) ;
#22539=DIRECTION ( 'NONE',  ( 1.000000000000000000, -0.000000000000000000, -0.000000000000000000 ) ) ;
#22600=EDGE_CURVE ( 'NONE', #55409, #27807, #71451, .T. ) ;
#22652=CYLINDRICAL_SURFACE ( 'NONE', #15533, 1.000000000000000888 ) ;
#22660=DIRECTION ( 'NONE',  ( 0.000000000000000000, 0.000000000000000000, 1.000000000000000000 ) ) ;
#22805=CARTESIAN_POINT ( 'NONE',  ( 143.6449502718966755, 0.000000000000000000, -47.19625681453479871 ) ) ;
#22831=VECTOR ( 'NONE', #68273, 1000.000000000000000 ) ;
#22833=DIRECTION ( 'NONE',  ( 0.000000000000000000, 0.000000000000000000, -1.000000000000000000 ) ) ;
#22864=ORIENTED_EDGE ( 'NONE', *, *, #6869, .F. ) ;
#22924=DIRECTION ( 'NONE',  ( -1.000000000000000000, -0.000000000000000000, -0.000000000000000000 ) ) ;
#23035=ADVANCED_FACE ( 'NONE', ( #83449 ), #33274, .T. ) ;
#23080=ORIENTED_EDGE ( 'NONE', *, *, #43751, .F. ) ;
#23090=AXIS2_PLACEMENT_3D ( 'NONE', #52721, #17225, #66045 ) ;
#23115=EDGE_CURVE ( 'NONE', #83756, #5915, #4922, .T. ) ;
#23162=CARTESIAN_POINT ( 'NONE',  ( 142.6449502718966755, -27.00396092263537540, 22.50000000000000000 ) ) ;
#23168=VECTOR ( 'NONE', #61126, 1000.000000000000114 ) ;
#23174=VECTOR ( 'NONE', #64807, 1000.000000000000000 ) ;
#23204=ORIENTED_EDGE ( 'NONE', *, *, #89909, .T. ) ;
#23207=LINE ( 'NONE', #37863, #20381 ) ;
#23230=AXIS2_PLACEMENT_3D ( 'NONE', #88800, #59017, #43856 ) ;
#23241=VERTEX_POINT ( 'NONE', #20004 ) ;
#23274=EDGE_CURVE ( 'NONE', #79714, #82047, #55999, .T. ) ;
#23279=AXIS2_PLACEMENT_3D ( 'NONE', #85409, #35215, #40879 ) ;
#23304=DIRECTION ( 'NONE',  ( 1.000000000000000000, 0.000000000000000000, 0.000000000000000000 ) ) ;
#23319=CIRCLE ( 'NONE', #53597, 1.000000000000000888 ) ;
#23321=CARTESIAN_POINT ( 'NONE',  ( -18.20453976106250948, -63.49190233628851132, -21.50000000000000000 ) ) ;
#23330=ADVANCED_FACE ( 'NONE', ( #46994 ), #26649, .F. ) ;
#23337=VECTOR ( 'NONE', #9557, 1000.000000000000000 ) ;
#23372=DIRECTION ( 'NONE',  ( -1.000000000000000000, 0.000000000000000000, 0.000000000000000000 ) ) ;
#23386=DIRECTION ( 'NONE',  ( 0.000000000000000000, 0.000000000000000000, 1.000000000000000000 ) ) ;
#23409=AXIS2_PLACEMENT_3D ( 'NONE', #71924, #85164, #86544 ) ;
#23454=ADVANCED_FACE ( 'NONE', ( #45711 ), #66594, .F. ) ;
#23483=CARTESIAN_POINT ( 'NONE',  ( 188.7399167944524550, -12.49482340714361506, 10.00000000000000000 ) ) ;
#23523=CYLINDRICAL_SURFACE ( 'NONE', #56248, 4.999999999999990230 ) ;
#23551=EDGE_LOOP ( 'NONE', ( #14876, #23699, #49436, #84236 ) ) ;
#23597=LINE ( 'NONE', #52464, #86857 ) ;
#23598=DIRECTION ( 'NONE',  ( -0.000000000000000000, -1.000000000000000000, -0.000000000000000000 ) ) ;
#23635=CARTESIAN_POINT ( 'NONE',  ( 60.29495240252359878, -249.1689065933675238, 21.50000000000000000 ) ) ;
#23683=VECTOR ( 'NONE', #37611, 1000.000000000000000 ) ;
#23692=ORIENTED_EDGE ( 'NONE', *, *, #86200, .T. ) ;
#23699=ORIENTED_EDGE ( 'NONE', *, *, #34031, .T. ) ;
#23719=CYLINDRICAL_SURFACE ( 'NONE', #83644, 1.000000000000000888 ) ;
#23741=CARTESIAN_POINT ( 'NONE',  ( 208.4306832106270804, -324.2391364535881735, 0.000000000000000000 ) ) ;
#23753=CARTESIAN_POINT ( 'NONE',  ( -23.68628624284178130, -44.55766379199612004, 21.50000000000000000 ) ) ;
#23782=CARTESIAN_POINT ( 'NONE',  ( 180.7149167944524493, -12.49482340714361506, 10.00000000000000000 ) ) ;
#23820=EDGE_LOOP ( 'NONE', ( #33566, #39244, #7536, #76828 ) ) ;
#23827=ORIENTED_EDGE ( 'NONE', *, *, #42791, .T. ) ;
#23828=DIRECTION ( 'NONE',  ( -0.000000000000000000, -0.000000000000000000, -1.000000000000000000 ) ) ;
#23831=ORIENTED_EDGE ( 'NONE', *, *, #87216, .F. ) ;
#23848=CARTESIAN_POINT ( 'NONE',  ( 184.7149167944524493, -12.49482340714361506, -3.999999999999998224 ) ) ;
#23881=LINE ( 'NONE', #71898, #17095 ) ;
#23920=AXIS2_PLACEMENT_3D ( 'NONE', #54514, #41220, #25632 ) ;
#23988=LINE ( 'NONE', #68957, #91232 ) ;
#24004=EDGE_LOOP ( 'NONE', ( #34502, #19347, #84806, #52128 ) ) ;
#24049=DIRECTION ( 'NONE',  ( -0.000000000000000000, -0.000000000000000000, 1.000000000000000000 ) ) ;
#24093=DIRECTION ( 'NONE',  ( 0.5335274993778010844, -0.8457827187922856149, 0.000000000000000000 ) ) ;
#24111=CIRCLE ( 'NONE', #89112, 1.000000000000000888 ) ;
#24118=CARTESIAN_POINT ( 'NONE',  ( 10.41963433625062230, -229.5268262511776527, 22.50000000000000000 ) ) ;
#24152=ORIENTED_EDGE ( 'NONE', *, *, #49321, .T. ) ;
#24174=EDGE_CURVE ( 'NONE', #72125, #40992, #93033, .T. ) ;
#24176=AXIS2_PLACEMENT_3D ( 'NONE', #42155, #55924, #42630 ) ;
#24236=AXIS2_PLACEMENT_3D ( 'NONE', #84201, #54854, #83736 ) ;
#24242=AXIS2_PLACEMENT_3D ( 'NONE', #5853, #91037, #26209 ) ;
#24257=EDGE_LOOP ( 'NONE', ( #45765, #85180, #47173, #19244 ) ) ;
#24290=ORIENTED_EDGE ( 'NONE', *, *, #73275, .F. ) ;
#24340=DIRECTION ( 'NONE',  ( -0.000000000000000000, 1.000000000000000000, 0.000000000000000000 ) ) ;
#24343=LINE ( 'NONE', #82099, #23174 ) ;
#24432=( LENGTH_UNIT ( ) NAMED_UNIT ( * ) SI_UNIT ( .MILLI., .METRE. ) );
#24445=AXIS2_PLACEMENT_3D ( 'NONE', #316, #78925, #29200 ) ;
#24481=EDGE_LOOP ( 'NONE', ( #19524, #61524, #78205, #44190 ) ) ;
#24506=ORIENTED_EDGE ( 'NONE', *, *, #84781, .F. ) ;
#24578=VECTOR ( 'NONE', #79317, 1000.000000000000000 ) ;
#24591=CIRCLE ( 'NONE', #29137, 12.68950434577434372 ) ;
#24599=DIRECTION ( 'NONE',  ( 0.8457827187922972723, 0.5335274993777825436, 0.000000000000000000 ) ) ;
#24610=EDGE_CURVE ( 'NONE', #67590, #26246, #32158, .T. ) ;
#24613=CIRCLE ( 'NONE', #11023, 1.000000000000002887 ) ;
#24617=AXIS2_PLACEMENT_3D ( 'NONE', #65961, #22833, #86294 ) ;
#24628=ORIENTED_EDGE ( 'NONE', *, *, #2847, .T. ) ;
#24661=AXIS2_PLACEMENT_3D ( 'NONE', #74732, #9853, #80894 ) ;
#24682=AXIS2_PLACEMENT_3D ( 'NONE', #88037, #46353, #75254 ) ;
#24714=FACE_OUTER_BOUND ( 'NONE', #77969, .T. ) ;
#24725=ADVANCED_FACE ( 'NONE', ( #46087 ), #37137, .F. ) ;
#24737=ORIENTED_EDGE ( 'NONE', *, *, #82544, .F. ) ;
#24744=( NAMED_UNIT ( * ) SI_UNIT ( $, .STERADIAN. ) SOLID_ANGLE_UNIT ( ) );
#24748=ORIENTED_EDGE ( 'NONE', *, *, #22475, .F. ) ;
#24780=CONICAL_SURFACE ( 'NONE', #23279, 4.025000000000000355, 0.7853981633973095011 ) ;
#24784=CARTESIAN_POINT ( 'NONE',  ( -23.68628624284178130, -43.55766379199612004, -22.50000000000000000 ) ) ;
#24820=LINE ( 'NONE', #67454, #31822 ) ;
#24828=AXIS2_PLACEMENT_3D ( 'NONE', #84098, #26350, #11668 ) ;
#24888=VECTOR ( 'NONE', #55365, 1000.000000000000000 ) ;
#24936=DIRECTION ( 'NONE',  ( -1.000000000000000000, 0.000000000000000000, 0.000000000000000000 ) ) ;
#24946=CIRCLE ( 'NONE', #43069, 160.1282194813176716 ) ;
#25042=DIRECTION ( 'NONE',  ( -0.8457827187922920542, -0.5335274993777912034, -0.000000000000000000 ) ) ;
#25101=ORIENTED_EDGE ( 'NONE', *, *, #10707, .T. ) ;
#25127=CARTESIAN_POINT ( 'NONE',  ( 223.4306832106270804, -135.2391364535880882, 21.50000000000000000 ) ) ;
#25139=DIRECTION ( 'NONE',  ( 1.124465274301078281E-16, 1.000000000000000000, -0.000000000000000000 ) ) ;
#25147=ADVANCED_FACE ( 'NONE', ( #31436 ), #17086, .T. ) ;
#25219=ORIENTED_EDGE ( 'NONE', *, *, #48693, .F. ) ;
#25263=DIRECTION ( 'NONE',  ( 0.000000000000000000, 0.000000000000000000, -1.000000000000000000 ) ) ;
#25276=ORIENTED_EDGE ( 'NONE', *, *, #4151, .F. ) ;
#25283=DIRECTION ( 'NONE',  ( 0.000000000000000000, 0.000000000000000000, 1.000000000000000000 ) ) ;
#25346=DIRECTION ( 'NONE',  ( 0.8571673007021122226, 0.000000000000000000, 0.5150380749100541555 ) ) ;
#25414=UNCERTAINTY_MEASURE_WITH_UNIT (LENGTH_MEASURE( 1.000000000000000082E-05 ), #24432, 'distance_accuracy_value', 'NONE');
#25446=FACE_OUTER_BOUND ( 'NONE', #86109, .T. ) ;
#25465=ADVANCED_FACE ( 'NONE', ( #19095 ), #3496, .F. ) ;
#25532=CIRCLE ( 'NONE', #27103, 203.9779373800640485 ) ;
#25535=DIRECTION ( 'NONE',  ( 8.659560562352529298E-17, 0.7071067811867438602, -0.7071067811863512853 ) ) ;
#25549=ADVANCED_FACE ( 'NONE', ( #46546 ), #38295, .T. ) ;
#25554=CARTESIAN_POINT ( 'NONE',  ( -36.09237171215955442, -55.96374926131388605, 21.50000000000000000 ) ) ;
#25569=ORIENTED_EDGE ( 'NONE', *, *, #68768, .T. ) ;
#25632=DIRECTION ( 'NONE',  ( 1.000000000000000000, -1.124465274301078034E-16, 0.000000000000000000 ) ) ;
#25794=VERTEX_POINT ( 'NONE', #41299 ) ;
#25799=AXIS2_PLACEMENT_3D ( 'NONE', #69303, #41328, #27152 ) ;
#25875=DIRECTION ( 'NONE',  ( 0.000000000000000000, 0.000000000000000000, 1.000000000000000000 ) ) ;
#25904=CARTESIAN_POINT ( 'NONE',  ( 221.8344101925596306, -44.55766379199612004, -21.50000000000000000 ) ) ;
#25920=EDGE_LOOP ( 'NONE', ( #76931, #20040, #69555, #28259 ) ) ;
#25922=LINE ( 'NONE', #83683, #65654 ) ;
#25940=VECTOR ( 'NONE', #19327, 1000.000000000000000 ) ;
#25953=DIRECTION ( 'NONE',  ( -1.000000000000000000, 0.000000000000000000, 0.000000000000000000 ) ) ;
#25970=VERTEX_POINT ( 'NONE', #13403 ) ;
#26007=ORIENTED_EDGE ( 'NONE', *, *, #13993, .F. ) ;
#26019=VERTEX_POINT ( 'NONE', #88004 ) ;
#26025=LINE ( 'NONE', #76232, #15832 ) ;
#26085=VERTEX_POINT ( 'NONE', #28081 ) ;
#26151=ORIENTED_EDGE ( 'NONE', *, *, #19791, .F. ) ;
#26165=DIRECTION ( 'NONE',  ( 0.000000000000000000, 0.000000000000000000, 1.000000000000000000 ) ) ;
#26206=AXIS2_PLACEMENT_3D ( 'NONE', #11835, #4734, #62520 ) ;
#26209=DIRECTION ( 'NONE',  ( 0.000000000000000000, -0.000000000000000000, -1.000000000000000000 ) ) ;
#26216=AXIS2_PLACEMENT_3D ( 'NONE', #7336, #5949, #5487 ) ;
#26244=AXIS2_PLACEMENT_3D ( 'NONE', #26462, #47751, #89906 ) ;
#26246=VERTEX_POINT ( 'NONE', #65831 ) ;
#26265=ORIENTED_EDGE ( 'NONE', *, *, #20409, .F. ) ;
#26275=VECTOR ( 'NONE', #14079, 1000.000000000000000 ) ;
#26287=LINE ( 'NONE', #68920, #70161 ) ;
#26299=VECTOR ( 'NONE', #76744, 1000.000000000000000 ) ;
#26316=DIRECTION ( 'NONE',  ( -0.000000000000000000, 1.000000000000000000, -0.000000000000000000 ) ) ;
#26350=DIRECTION ( 'NONE',  ( -0.000000000000000000, -0.000000000000000000, -1.000000000000000000 ) ) ;
#26366=TOROIDAL_SURFACE ( 'NONE', #85299, 8.222204860432958284, 1.000000000000000000 ) ;
#26408=ORIENTED_EDGE ( 'NONE', *, *, #23274, .F. ) ;
#26424=PLANE ( 'NONE',  #47330 ) ;
#26462=CARTESIAN_POINT ( 'NONE',  ( 17.06571399127465583, -89.54582641780471874, 22.50000000000000000 ) ) ;
#26494=VERTEX_POINT ( 'NONE', #16070 ) ;
#26543=EDGE_CURVE ( 'NONE', #61209, #83756, #82162, .T. ) ;
#26571=CARTESIAN_POINT ( 'NONE',  ( 195.7510731661265595, -142.7221692137691775, -32.50000000000000711 ) ) ;
#26584=DIRECTION ( 'NONE',  ( -0.000000000000000000, -0.000000000000000000, -1.000000000000000000 ) ) ;
#26649=CYLINDRICAL_SURFACE ( 'NONE', #72991, 4.000000000000003553 ) ;
#26693=DIRECTION ( 'NONE',  ( -0.5335274993777934238, 0.8457827187922903889, 0.000000000000000000 ) ) ;
#26815=ADVANCED_FACE ( 'NONE', ( #61500 ), #60561, .T. ) ;
#26874=PLANE ( 'NONE',  #64107 ) ;
#26903=DIRECTION ( 'NONE',  ( -0.000000000000000000, -0.000000000000000000, -1.000000000000000000 ) ) ;
#26950=DIRECTION ( 'NONE',  ( 1.000000000000000000, 0.000000000000000000, 0.000000000000000000 ) ) ;
#26979=EDGE_CURVE ( 'NONE', #37428, #70302, #12504, .T. ) ;
#26987=EDGE_LOOP ( 'NONE', ( #89711, #93376, #71721, #80635 ) ) ;
#27050=CARTESIAN_POINT ( 'NONE',  ( 194.5881128153457098, 0.000000000000000000, 21.50000000000000000 ) ) ;
#27088=ORIENTED_EDGE ( 'NONE', *, *, #42244, .T. ) ;
#27096=CARTESIAN_POINT ( 'NONE',  ( 165.2494399300530290, -11.64849832608277325, -6.403442476110241977 ) ) ;
#27103=AXIS2_PLACEMENT_3D ( 'NONE', #22354, #13874, #72112 ) ;
#27120=EDGE_CURVE ( 'NONE', #93680, #28617, #81263, .T. ) ;
#27127=DIRECTION ( 'NONE',  ( 0.000000000000000000, 0.000000000000000000, -1.000000000000000000 ) ) ;
#27152=DIRECTION ( 'NONE',  ( 0.000000000000000000, 0.000000000000000000, 1.000000000000000000 ) ) ;
#27196=EDGE_CURVE ( 'NONE', #4433, #78431, #53314, .T. ) ;
#27238=CARTESIAN_POINT ( 'NONE',  ( 161.2494399300530290, -11.64849832608277325, 10.00000000000000000 ) ) ;
#27246=MANIFOLD_SOLID_BREP ( 'Fillet17', #12891 ) ;
#27308=LINE ( 'NONE', #70418, #6653 ) ;
#27327=ORIENTED_EDGE ( 'NONE', *, *, #69069, .T. ) ;
#27329=DIRECTION ( 'NONE',  ( -1.000000000000000000, 0.000000000000000000, 0.000000000000000000 ) ) ;
#27341=ORIENTED_EDGE ( 'NONE', *, *, #86916, .T. ) ;
#27342=ORIENTED_EDGE ( 'NONE', *, *, #87285, .F. ) ;
#27345=EDGE_CURVE ( 'NONE', #72125, #79604, #45719, .T. ) ;
#27371=CARTESIAN_POINT ( 'NONE',  ( 196.7510731661265595, -143.7221692137691775, 21.50000000000000000 ) ) ;
#27393=ORIENTED_EDGE ( 'NONE', *, *, #16696, .F. ) ;
#27465=DIRECTION ( 'NONE',  ( -1.000000000000000000, 0.000000000000000000, -0.000000000000000000 ) ) ;
#27505=EDGE_LOOP ( 'NONE', ( #83633, #29187, #57722, #52742 ) ) ;
#27506=CARTESIAN_POINT ( 'NONE',  ( 143.6449502718966755, 0.000000000000000000, 21.50000000000000000 ) ) ;
#27509=CARTESIAN_POINT ( 'NONE',  ( 143.6449502718966755, -26.00396092263537895, 22.08578643762690419 ) ) ;
#27512=EDGE_CURVE ( 'NONE', #4350, #25794, #33404, .T. ) ;
#27513=EDGE_CURVE ( 'NONE', #21234, #61209, #42707, .T. ) ;
#27538=ORIENTED_EDGE ( 'NONE', *, *, #45025, .F. ) ;
#27582=TOROIDAL_SURFACE ( 'NONE', #38149, 16.36528803885689243, 1.000000000000000000 ) ;
#27685=ORIENTED_EDGE ( 'NONE', *, *, #38265, .T. ) ;
#27726=DIRECTION ( 'NONE',  ( 0.000000000000000000, 0.000000000000000000, 1.000000000000000000 ) ) ;
#27744=DIRECTION ( 'NONE',  ( 0.000000000000000000, 0.5150380749100592626, 0.8571673007021092250 ) ) ;
#27776=EDGE_LOOP ( 'NONE', ( #3700, #12399, #30680 ) ) ;
#27777=ORIENTED_EDGE ( 'NONE', *, *, #90893, .T. ) ;
#27780=AXIS2_PLACEMENT_3D ( 'NONE', #88358, #59508, #88814 ) ;
#27807=VERTEX_POINT ( 'NONE', #57893 ) ;
#27883=AXIS2_PLACEMENT_3D ( 'NONE', #82418, #30844, #9975 ) ;
#27910=CYLINDRICAL_SURFACE ( 'NONE', #58242, 1.000000000000000888 ) ;
#27960=DIRECTION ( 'NONE',  ( -0.000000000000000000, 1.000000000000000000, 0.000000000000000000 ) ) ;
#27992=ORIENTED_EDGE ( 'NONE', *, *, #72204, .F. ) ;
#28033=ORIENTED_EDGE ( 'NONE', *, *, #53026, .T. ) ;
#28081=CARTESIAN_POINT ( 'NONE',  ( 223.4306832106270804, -135.2391364535880882, -21.50000000000000000 ) ) ;
#28235=AXIS2_PLACEMENT_3D ( 'NONE', #73765, #88877, #72831 ) ;
#28259=ORIENTED_EDGE ( 'NONE', *, *, #2228, .T. ) ;
#28267=ORIENTED_EDGE ( 'NONE', *, *, #940, .T. ) ;
#28272=CARTESIAN_POINT ( 'NONE',  ( 222.4201966301864672, -44.14345022962302068, -22.50000000000000000 ) ) ;
#28314=DIRECTION ( 'NONE',  ( -1.224646799147353207E-16, 1.000000000000000000, 0.000000000000000000 ) ) ;
#28351=ORIENTED_EDGE ( 'NONE', *, *, #60229, .F. ) ;
#28365=CARTESIAN_POINT ( 'NONE',  ( 165.2494399300530290, -11.64849832608277325, 9.974999999999996092 ) ) ;
#28426=CARTESIAN_POINT ( 'NONE',  ( 73.43068321062709458, -134.2391364535880598, -4.999999999999990230 ) ) ;
#28478=ORIENTED_EDGE ( 'NONE', *, *, #62997, .T. ) ;
#28542=DIRECTION ( 'NONE',  ( 0.000000000000000000, 0.000000000000000000, 1.000000000000000000 ) ) ;
#28544=CARTESIAN_POINT ( 'NONE',  ( 195.7510731661265595, -142.7221692137691775, -21.50000000000000000 ) ) ;
#28588=EDGE_CURVE ( 'NONE', #37463, #68679, #29198, .T. ) ;
#28595=ORIENTED_EDGE ( 'NONE', *, *, #6798, .F. ) ;
#28617=VERTEX_POINT ( 'NONE', #23753 ) ;
#28623=ORIENTED_EDGE ( 'NONE', *, *, #44041, .F. ) ;
#28665=AXIS2_PLACEMENT_3D ( 'NONE', #81508, #9541, #16655 ) ;
#28728=CARTESIAN_POINT ( 'NONE',  ( 221.8344101925596306, -0.9999999999999991118, 22.50000000000000000 ) ) ;
#28731=TOROIDAL_SURFACE ( 'NONE', #18101, 203.9779373800640485, 1.000000000000000000 ) ;
#28739=CARTESIAN_POINT ( 'NONE',  ( 10.19742947581765691, -229.5268262511776527, 22.50000000000000000 ) ) ;
#28745=FACE_OUTER_BOUND ( 'NONE', #7274, .T. ) ;
#28775=DIRECTION ( 'NONE',  ( -0.7071067811864494290, 8.659560562353731078E-17, 0.7071067811866457165 ) ) ;
#28803=CARTESIAN_POINT ( 'NONE',  ( -23.68628624284178130, -55.96374926131388605, 22.50000000000000000 ) ) ;
#28827=LINE ( 'NONE', #20785, #92963 ) ;
#28909=EDGE_CURVE ( 'NONE', #17995, #46866, #9057, .T. ) ;
#28926=SPHERICAL_SURFACE ( 'NONE', #30915, 1.000000000000000000 ) ;
#28931=AXIS2_PLACEMENT_3D ( 'NONE', #13448, #42298, #19593 ) ;
#28968=ORIENTED_EDGE ( 'NONE', *, *, #13331, .T. ) ;
#28994=DIRECTION ( 'NONE',  ( -0.000000000000000000, 0.000000000000000000, 1.000000000000000000 ) ) ;
#29017=VERTEX_POINT ( 'NONE', #32728 ) ;
#29100=CARTESIAN_POINT ( 'NONE',  ( 165.2494399300530290, -11.64849832608277325, -3.999999999999998224 ) ) ;
#29137=AXIS2_PLACEMENT_3D ( 'NONE', #77058, #41030, #63350 ) ;
#29162=AXIS2_PLACEMENT_3D ( 'NONE', #78292, #43678, #614 ) ;
#29187=ORIENTED_EDGE ( 'NONE', *, *, #38462, .T. ) ;
#29198=CIRCLE ( 'NONE', #3430, 1.000000000000000888 ) ;
#29200=DIRECTION ( 'NONE',  ( 0.000000000000000000, 0.000000000000000000, -1.000000000000000000 ) ) ;
#29222=EDGE_CURVE ( 'NONE', #61220, #18301, #4307, .T. ) ;
#29224=CYLINDRICAL_SURFACE ( 'NONE', #42830, 0.9999999999999954481 ) ;
#29264=VERTEX_POINT ( 'NONE', #54488 ) ;
#29273=VECTOR ( 'NONE', #88118, 1000.000000000000000 ) ;
#29283=CIRCLE ( 'NONE', #41345, 7.500000000000007105 ) ;
#29328=VERTEX_POINT ( 'NONE', #62075 ) ;
#29348=FACE_OUTER_BOUND ( 'NONE', #52071, .T. ) ;
#29385=LINE ( 'NONE', #36474, #92748 ) ;
#29416=CIRCLE ( 'NONE', #89879, 4.999999999999990230 ) ;
#29436=AXIS2_PLACEMENT_3D ( 'NONE', #69100, #84217, #18910 ) ;
#29483=DIRECTION ( 'NONE',  ( 1.000000000000000000, 0.000000000000000000, 0.000000000000000000 ) ) ;
#29490=AXIS2_PLACEMENT_3D ( 'NONE', #31742, #75758, #33137 ) ;
#29534=ORIENTED_EDGE ( 'NONE', *, *, #77089, .F. ) ;
#29537=ADVANCED_FACE ( 'NONE', ( #44894 ), #8911, .T. ) ;
#29553=ORIENTED_EDGE ( 'NONE', *, *, #940, .F. ) ;
#29577=VECTOR ( 'NONE', #43389, 1000.000000000000000 ) ;
#29610=FACE_OUTER_BOUND ( 'NONE', #92635, .T. ) ;
#29666=ORIENTED_EDGE ( 'NONE', *, *, #50363, .T. ) ;
#29712=CARTESIAN_POINT ( 'NONE',  ( -47.80257052418233599, -229.5268262511776527, -22.50000000000000000 ) ) ;
#29734=ORIENTED_EDGE ( 'NONE', *, *, #79978, .F. ) ;
#29763=EDGE_CURVE ( 'NONE', #46033, #41118, #65521, .T. ) ;
#29793=ORIENTED_EDGE ( 'NONE', *, *, #91737, .T. ) ;
#29809=CARTESIAN_POINT ( 'NONE',  ( -35.09237171215954021, -122.5496321078137356, 22.50000000000000000 ) ) ;
#29844=FACE_OUTER_BOUND ( 'NONE', #50121, .T. ) ;
#29947=CIRCLE ( 'NONE', #90396, 1.000000000000000888 ) ;
#30013=EDGE_LOOP ( 'NONE', ( #39926, #76600, #28267, #82621 ) ) ;
#30080=VECTOR ( 'NONE', #79666, 1000.000000000000000 ) ;
#30127=DIRECTION ( 'NONE',  ( 0.8043439146810367202, -0.5941640067486294585, 0.000000000000000000 ) ) ;
#30132=VERTEX_POINT ( 'NONE', #90305 ) ;
#30169=CARTESIAN_POINT ( 'NONE',  ( 196.7510731661265595, -143.7221692137691775, -21.50000000000000000 ) ) ;
#30188=DIRECTION ( 'NONE',  ( -1.000000000000000000, 0.000000000000000000, 0.000000000000000000 ) ) ;
#30197=EDGE_LOOP ( 'NONE', ( #651, #59016, #54294, #23827, #43680, #48630, #47382, #8540, #20080, #57259, #51084, #10971, #68501, #39872, #27777, #12663, #6827, #35334 ) ) ;
#30206=AXIS2_PLACEMENT_3D ( 'NONE', #3858, #83369, #89533 ) ;
#30274=CIRCLE ( 'NONE', #24236, 7.999999999999992895 ) ;
#30275=DIRECTION ( 'NONE',  ( -0.000000000000000000, -0.000000000000000000, -1.000000000000000000 ) ) ;
#30285=EDGE_CURVE ( 'NONE', #77294, #26019, #62313, .T. ) ;
#30379=CARTESIAN_POINT ( 'NONE',  ( 195.5881128153457098, 15.36528803885690664, 22.50000000000000000 ) ) ;
#30421=FACE_OUTER_BOUND ( 'NONE', #34325, .T. ) ;
#30489=DIRECTION ( 'NONE',  ( 0.000000000000000000, 0.000000000000000000, 1.000000000000000000 ) ) ;
#30492=EDGE_CURVE ( 'NONE', #51697, #17995, #6033, .T. ) ;
#30515=ORIENTED_EDGE ( 'NONE', *, *, #5090, .T. ) ;
#30541=VECTOR ( 'NONE', #39321, 1000.000000000000000 ) ;
#30561=CARTESIAN_POINT ( 'NONE',  ( -23.40286736638519471, -134.2391364535880598, 21.50000000000000000 ) ) ;
#30606=DIRECTION ( 'NONE',  ( -0.000000000000000000, 1.000000000000000000, -0.000000000000000000 ) ) ;
#30623=CARTESIAN_POINT ( 'NONE',  ( 123.4306832106270946, -134.2391364535880882, -5.024999999999987921 ) ) ;
#30662=ORIENTED_EDGE ( 'NONE', *, *, #48158, .F. ) ;
#30680=ORIENTED_EDGE ( 'NONE', *, *, #18534, .F. ) ;
#30731=CARTESIAN_POINT ( 'NONE',  ( -47.80257052418233599, -229.5268262511776527, 22.47499999999998721 ) ) ;
#30765=AXIS2_PLACEMENT_3D ( 'NONE', #22805, #51672, #28994 ) ;
#30767=EDGE_CURVE ( 'NONE', #22436, #14651, #13150, .T. ) ;
#30789=DIRECTION ( 'NONE',  ( -0.000000000000000000, -0.000000000000000000, 1.000000000000000000 ) ) ;
#30831=VERTEX_POINT ( 'NONE', #57623 ) ;
#30836=CIRCLE ( 'NONE', #88261, 7.500000000000007105 ) ;
#30844=DIRECTION ( 'NONE',  ( 0.000000000000000000, 1.000000000000000000, 0.000000000000000000 ) ) ;
#30845=CIRCLE ( 'NONE', #80705, 1.000000000000003331 ) ;
#30881=FACE_OUTER_BOUND ( 'NONE', #87287, .T. ) ;
#30915=AXIS2_PLACEMENT_3D ( 'NONE', #13794, #42646, #6218 ) ;
#30918=ORIENTED_EDGE ( 'NONE', *, *, #86831, .T. ) ;
#30970=CARTESIAN_POINT ( 'NONE',  ( 139.6925840978351516, 15.36528803885690664, -21.50000000000000000 ) ) ;
#30987=CYLINDRICAL_SURFACE ( 'NONE', #89045, 1.000000000000000888 ) ;
#31096=CARTESIAN_POINT ( 'NONE',  ( 221.8344101925596306, -44.55766379199612004, -22.50000000000000000 ) ) ;
#31115=CARTESIAN_POINT ( 'NONE',  ( 60.29495240252359878, -249.1689065933675238, 22.50000000000000000 ) ) ;
#31144=DIRECTION ( 'NONE',  ( 0.7071067811864494290, 0.000000000000000000, 0.7071067811866457165 ) ) ;
#31155=LINE ( 'NONE', #88878, #83872 ) ;
#31192=ORIENTED_EDGE ( 'NONE', *, *, #60666, .T. ) ;
#31256=DIRECTION ( 'NONE',  ( -0.000000000000000000, -1.000000000000000000, -0.000000000000000000 ) ) ;
#31258=DIRECTION ( 'NONE',  ( -0.000000000000000000, -1.000000000000000000, -0.000000000000000000 ) ) ;
#31262=DIRECTION ( 'NONE',  ( 1.000000000000000000, -0.000000000000000000, -0.000000000000000000 ) ) ;
#31310=CARTESIAN_POINT ( 'NONE',  ( 194.5881128153457098, -26.00396092263537540, 21.50000000000000000 ) ) ;
#31362=LINE ( 'NONE', #81526, #57664 ) ;
#31376=ORIENTED_EDGE ( 'NONE', *, *, #54639, .F. ) ;
#31379=ORIENTED_EDGE ( 'NONE', *, *, #14648, .T. ) ;
#31405=EDGE_CURVE ( 'NONE', #26494, #44526, #270, .T. ) ;
#31436=FACE_OUTER_BOUND ( 'NONE', #3635, .T. ) ;
#31503=VECTOR ( 'NONE', #14274, 1000.000000000000000 ) ;
#31525=DIRECTION ( 'NONE',  ( -0.000000000000000000, -0.000000000000000000, 1.000000000000000000 ) ) ;
#31531=DIRECTION ( 'NONE',  ( -0.000000000000000000, -0.000000000000000000, -1.000000000000000000 ) ) ;
#31553=CARTESIAN_POINT ( 'NONE',  ( -23.68628624284178130, -44.55766379199612004, 21.50000000000000000 ) ) ;
#31645=ORIENTED_EDGE ( 'NONE', *, *, #9205, .F. ) ;
#31715=CARTESIAN_POINT ( 'NONE',  ( 208.4306832106271088, 42.44233620800392970, -7.500000000000012434 ) ) ;
#31716=ORIENTED_EDGE ( 'NONE', *, *, #10707, .F. ) ;
#31728=EDGE_LOOP ( 'NONE', ( #19512, #37845, #93570, #56816 ) ) ;
#31742=CARTESIAN_POINT ( 'NONE',  ( 73.43068321062709458, -134.2641364535880939, 0.000000000000000000 ) ) ;
#31755=FACE_OUTER_BOUND ( 'NONE', #70860, .T. ) ;
#31760=CIRCLE ( 'NONE', #24176, 4.999999999999990230 ) ;
#31797=EDGE_CURVE ( 'NONE', #46866, #44867, #47464, .T. ) ;
#31800=DIRECTION ( 'NONE',  ( 0.000000000000000000, 0.000000000000000000, 1.000000000000000000 ) ) ;
#31819=CARTESIAN_POINT ( 'NONE',  ( 17.06571399127465583, -89.54582641780471874, 22.50000000000000000 ) ) ;
#31822=VECTOR ( 'NONE', #81628, 1000.000000000000000 ) ;
#31843=DIRECTION ( 'NONE',  ( 0.000000000000000000, 0.000000000000000000, 1.000000000000000000 ) ) ;
#31859=ORIENTED_EDGE ( 'NONE', *, *, #51756, .F. ) ;
#31870=ADVANCED_FACE ( 'NONE', ( #77301 ), #56615, .T. ) ;
#31883=DIRECTION ( 'NONE',  ( -1.000000000000000000, 0.000000000000000000, 0.000000000000000000 ) ) ;
#31893=DIRECTION ( 'NONE',  ( -1.000000000000000000, 0.000000000000000000, 0.000000000000000000 ) ) ;
#31917=DIRECTION ( 'NONE',  ( -1.000000000000000000, 1.124465274301078034E-16, 0.000000000000000000 ) ) ;
#31920=DIRECTION ( 'NONE',  ( -1.000000000000000000, -9.031908658476993102E-16, 0.000000000000000000 ) ) ;
#31952=ORIENTED_EDGE ( 'NONE', *, *, #63462, .T. ) ;
#31981=CARTESIAN_POINT ( 'NONE',  ( 222.8344101925596306, -44.55766379199612004, 22.50000000000000000 ) ) ;
#32017=CARTESIAN_POINT ( 'NONE',  ( -35.09237171215954731, -55.96374926131388605, 22.50000000000000000 ) ) ;
#32030=DIRECTION ( 'NONE',  ( 1.000000000000000000, 0.000000000000000000, 0.000000000000000000 ) ) ;
#32091=AXIS2_PLACEMENT_3D ( 'NONE', #60315, #10556, #31883 ) ;
#32100=EDGE_CURVE ( 'NONE', #82047, #58642, #77747, .T. ) ;
#32158=CIRCLE ( 'NONE', #10982, 2.000000000000001776 ) ;
#32169=VECTOR ( 'NONE', #78468, 1000.000000000000000 ) ;
#32325=DIRECTION ( 'NONE',  ( -0.8571673007021122226, 1.049727191138618696E-16, 0.5150380749100541555 ) ) ;
#32334=CIRCLE ( 'NONE', #5102, 2.000000000000001776 ) ;
#32376=CARTESIAN_POINT ( 'NONE',  ( 139.6925840978351516, -141.7221692137691775, 21.50000000000000000 ) ) ;
#32391=AXIS2_PLACEMENT_3D ( 'NONE', #6752, #66365, #86250 ) ;
#32413=CARTESIAN_POINT ( 'NONE',  ( 208.4306832106271088, -44.55766379199612004, 0.000000000000000000 ) ) ;
#32468=ADVANCED_FACE ( 'NONE', ( #8123 ), #22333, .T. ) ;
#32495=DIRECTION ( 'NONE',  ( 0.000000000000000000, 0.000000000000000000, -1.000000000000000000 ) ) ;
#32540=CIRCLE ( 'NONE', #88481, 4.000000000000003553 ) ;
#32648=VERTEX_POINT ( 'NONE', #25127 ) ;
#32683=CARTESIAN_POINT ( 'NONE',  ( -18.20453976106250948, -63.49190233628851132, -22.50000000000000000 ) ) ;
#32726=DIRECTION ( 'NONE',  ( -1.000000000000000000, 0.000000000000000000, 0.000000000000000000 ) ) ;
#32728=CARTESIAN_POINT ( 'NONE',  ( 208.4306832106271088, 0.000000000000000000, -7.500000000000012434 ) ) ;
#32737=EDGE_LOOP ( 'NONE', ( #48032, #60302, #85533, #83482 ) ) ;
#32753=CARTESIAN_POINT ( 'NONE',  ( -35.09237171215954731, -122.5496321078137356, 21.50000000000000000 ) ) ;
#32768=ORIENTED_EDGE ( 'NONE', *, *, #62017, .F. ) ;
#32770=ORIENTED_EDGE ( 'NONE', *, *, #27512, .T. ) ;
#32853=VERTEX_POINT ( 'NONE', #37911 ) ;
#32868=ADVANCED_FACE ( 'NONE', ( #60194 ), #68690, .T. ) ;
#32888=ORIENTED_EDGE ( 'NONE', *, *, #43122, .T. ) ;
#33015=ORIENTED_EDGE ( 'NONE', *, *, #53026, .F. ) ;
#33066=DIRECTION ( 'NONE',  ( -0.4467993836324651857, 0.8946341770721982778, 0.000000000000000000 ) ) ;
#33103=CARTESIAN_POINT ( 'NONE',  ( 143.6449502718966755, 0.000000000000000000, -47.19625681453479871 ) ) ;
#33113=DIRECTION ( 'NONE',  ( -0.000000000000000000, 1.000000000000000000, -0.000000000000000000 ) ) ;
#33137=DIRECTION ( 'NONE',  ( 0.000000000000000000, 0.000000000000000000, 1.000000000000000000 ) ) ;
#33168=LINE ( 'NONE', #55432, #61119 ) ;
#33211=DIRECTION ( 'NONE',  ( 0.000000000000000000, 0.000000000000000000, 1.000000000000000000 ) ) ;
#33250=ORIENTED_EDGE ( 'NONE', *, *, #87501, .T. ) ;
#33274=SPHERICAL_SURFACE ( 'NONE', #39690, 1.000000000000000000 ) ;
#33278=EDGE_CURVE ( 'NONE', #79714, #50388, #58090, .T. ) ;
#33292=VERTEX_POINT ( 'NONE', #83331 ) ;
#33311=PLANE ( 'NONE',  #24242 ) ;
#33379=EDGE_CURVE ( 'NONE', #46977, #37463, #59652, .T. ) ;
#33383=CARTESIAN_POINT ( 'NONE',  ( 196.7510731661265595, -141.7221692137691775, 22.50000000000000000 ) ) ;
#33404=LINE ( 'NONE', #5005, #48715 ) ;
#33410=LINE ( 'NONE', #12106, #19932 ) ;
#33417=PLANE ( 'NONE',  #7625 ) ;
#33548=DIRECTION ( 'NONE',  ( -0.000000000000000000, -0.000000000000000000, 1.000000000000000000 ) ) ;
#33566=ORIENTED_EDGE ( 'NONE', *, *, #78869, .F. ) ;
#33571=CARTESIAN_POINT ( 'NONE',  ( -18.20453976106250948, -63.49190233628851132, 22.50000000000000000 ) ) ;
#33646=AXIS2_PLACEMENT_3D ( 'NONE', #75225, #10339, #89876 ) ;
#33679=LINE ( 'NONE', #32753, #65681 ) ;
#33703=DIRECTION ( 'NONE',  ( 1.000000000000000000, 0.000000000000000000, 0.000000000000000000 ) ) ;
#33716=CARTESIAN_POINT ( 'NONE',  ( 196.7510731661265595, -143.7221692137691775, -21.50000000000000000 ) ) ;
#33733=CIRCLE ( 'NONE', #9511, 8.000000000000000000 ) ;
#33808=CARTESIAN_POINT ( 'NONE',  ( -39.80257052418234309, -229.5268262511776527, -22.50000000000000000 ) ) ;
#33867=AXIS2_PLACEMENT_3D ( 'NONE', #18392, #68596, #82782 ) ;
#33885=CARTESIAN_POINT ( 'NONE',  ( 194.5881128153457098, -26.00396092263537540, 21.50000000000000000 ) ) ;
#33922=CIRCLE ( 'NONE', #45995, 4.000000000000003553 ) ;
#33969=FACE_OUTER_BOUND ( 'NONE', #72818, .T. ) ;
#33977=CARTESIAN_POINT ( 'NONE',  ( 222.8344101925596306, 0.000000000000000000, -21.49999999999998579 ) ) ;
#34031=EDGE_CURVE ( 'NONE', #12908, #48629, #23597, .T. ) ;
#34073=VERTEX_POINT ( 'NONE', #67624 ) ;
#34074=EDGE_CURVE ( 'NONE', #58890, #63355, #11078, .T. ) ;
#34096=AXIS2_PLACEMENT_3D ( 'NONE', #25904, #91227, #60988 ) ;
#34149=DIRECTION ( 'NONE',  ( 0.5941640067486159138, -0.8043439146810467122, 0.000000000000000000 ) ) ;
#34164=DIRECTION ( 'NONE',  ( 1.000000000000000000, -0.000000000000000000, 0.000000000000000000 ) ) ;
#34325=EDGE_LOOP ( 'NONE', ( #31192, #26007, #64112, #19045 ) ) ;
#34350=EDGE_CURVE ( 'NONE', #57488, #89567, #38247, .T. ) ;
#34404=ORIENTED_EDGE ( 'NONE', *, *, #87492, .F. ) ;
#34428=EDGE_CURVE ( 'NONE', #72836, #76418, #33733, .T. ) ;
#34502=ORIENTED_EDGE ( 'NONE', *, *, #68908, .T. ) ;
#34611=DIRECTION ( 'NONE',  ( -0.5335274993777825436, 0.8457827187922972723, 0.000000000000000000 ) ) ;
#34662=ORIENTED_EDGE ( 'NONE', *, *, #37291, .T. ) ;
#34673=EDGE_CURVE ( 'NONE', #55168, #72836, #65699, .T. ) ;
#34817=CARTESIAN_POINT ( 'NONE',  ( 208.4306832106271088, -142.7221692137691775, 0.000000000000000000 ) ) ;
#34876=DIRECTION ( 'NONE',  ( 1.124465274301078034E-16, 1.000000000000000000, 0.000000000000000000 ) ) ;
#34897=LINE ( 'NONE', #85548, #21929 ) ;
#34904=FACE_OUTER_BOUND ( 'NONE', #88431, .T. ) ;
#34962=ORIENTED_EDGE ( 'NONE', *, *, #66220, .F. ) ;
#35007=AXIS2_PLACEMENT_3D ( 'NONE', #70971, #5641, #6578 ) ;
#35038=CARTESIAN_POINT ( 'NONE',  ( -187.9122233887894140, -89.54582641780471874, -21.50000000000000000 ) ) ;
#35039=SPHERICAL_SURFACE ( 'NONE', #4982, 1.000000000000000000 ) ;
#35078=AXIS2_PLACEMENT_3D ( 'NONE', #27371, #20736, #56261 ) ;
#35088=LINE ( 'NONE', #78655, #31503 ) ;
#35185=FACE_OUTER_BOUND ( 'NONE', #4716, .T. ) ;
#35215=DIRECTION ( 'NONE',  ( -0.000000000000000000, -0.000000000000000000, 1.000000000000000000 ) ) ;
#35245=AXIS2_PLACEMENT_3D ( 'NONE', #71691, #31262, #9453 ) ;
#35252=ORIENTED_EDGE ( 'NONE', *, *, #90641, .T. ) ;
#35274=AXIS2_PLACEMENT_3D ( 'NONE', #39431, #11034, #31893 ) ;
#35334=ORIENTED_EDGE ( 'NONE', *, *, #7047, .T. ) ;
#35347=CARTESIAN_POINT ( 'NONE',  ( 208.4306832106271088, -134.2391364535880882, 0.000000000000000000 ) ) ;
#35368=DIRECTION ( 'NONE',  ( -0.000000000000000000, -0.000000000000000000, 1.000000000000000000 ) ) ;
#35373=AXIS2_PLACEMENT_3D ( 'NONE', #85106, #78945, #5591 ) ;
#35416=CYLINDRICAL_SURFACE ( 'NONE', #79310, 7.999999999999992895 ) ;
#35435=VECTOR ( 'NONE', #64907, 1000.000000000000000 ) ;
#35504=EDGE_LOOP ( 'NONE', ( #11454, #47572, #23204, #34662 ) ) ;
#35506=DIRECTION ( 'NONE',  ( -0.000000000000000000, 1.000000000000000000, -0.000000000000000000 ) ) ;
#35535=CARTESIAN_POINT ( 'NONE',  ( 17.06571399127465583, -89.54582641780471874, -21.50000000000000000 ) ) ;
#35541=EDGE_CURVE ( 'NONE', #41591, #61220, #42854, .T. ) ;
#35576=CONICAL_SURFACE ( 'NONE', #41562, 4.999999999999990230, 1.029744258676656754 ) ;
#35601=DIRECTION ( 'NONE',  ( -0.000000000000000000, -0.000000000000000000, 1.000000000000000000 ) ) ;
#35648=LINE ( 'NONE', #85813, #69544 ) ;
#35651=AXIS2_PLACEMENT_3D ( 'NONE', #92172, #20695, #27329 ) ;
#35671=ORIENTED_EDGE ( 'NONE', *, *, #38515, .T. ) ;
#35724=VECTOR ( 'NONE', #16930, 1000.000000000000000 ) ;
#35740=DIRECTION ( 'NONE',  ( -0.000000000000000000, -0.000000000000000000, -1.000000000000000000 ) ) ;
#35829=ORIENTED_EDGE ( 'NONE', *, *, #5207, .T. ) ;
#35832=CARTESIAN_POINT ( 'NONE',  ( 139.6925840978351516, 15.36528803885690664, 22.50000000000000000 ) ) ;
#35915=CARTESIAN_POINT ( 'NONE',  ( 165.2494399300530290, -11.64849832608277325, -3.999999999999998224 ) ) ;
#36009=ADVANCED_FACE ( 'NONE', ( #36094 ), #114, .F. ) ;
#36050=EDGE_LOOP ( 'NONE', ( #8235, #79842, #37979, #3189 ) ) ;
#36068=ORIENTED_EDGE ( 'NONE', *, *, #54005, .F. ) ;
#36094=FACE_OUTER_BOUND ( 'NONE', #32737, .T. ) ;
#36226=VECTOR ( 'NONE', #78272, 1000.000000000000000 ) ;
#36269=CARTESIAN_POINT ( 'NONE',  ( 188.7149167944524493, -12.49482340714361506, -3.999999999999998224 ) ) ;
#36284=ORIENTED_EDGE ( 'NONE', *, *, #75213, .F. ) ;
#36314=ADVANCED_FACE ( 'NONE', ( #60207 ), #82882, .F. ) ;
#36318=PLANE ( 'NONE',  #73123 ) ;
#36359=DIRECTION ( 'NONE',  ( -1.000000000000000000, 8.928268813181216143E-16, 0.000000000000000000 ) ) ;
#36404=ADVANCED_FACE ( 'NONE', ( #88592 ), #16633, .F. ) ;
#36437=LINE ( 'NONE', #13282, #501 ) ;
#36474=CARTESIAN_POINT ( 'NONE',  ( 222.8344101925596306, 0.000000000000000000, 22.50000000000000000 ) ) ;
#36509=ORIENTED_EDGE ( 'NONE', *, *, #37177, .T. ) ;
#36757=FACE_OUTER_BOUND ( 'NONE', #65310, .T. ) ;
#36780=DIRECTION ( 'NONE',  ( -0.000000000000000000, -0.000000000000000000, 1.000000000000000000 ) ) ;
#36888=ORIENTED_EDGE ( 'NONE', *, *, #42791, .F. ) ;
#36914=CIRCLE ( 'NONE', #64195, 16.36528803885689598 ) ;
#36924=AXIS2_PLACEMENT_3D ( 'NONE', #69727, #6271, #26165 ) ;
#36985=CARTESIAN_POINT ( 'NONE',  ( 222.4306832106270804, -141.7221692137691775, 21.50000000000000000 ) ) ;
#37045=EDGE_LOOP ( 'NONE', ( #48702, #47761, #19120 ) ) ;
#37137=CYLINDRICAL_SURFACE ( 'NONE', #23090, 11.68950434577434372 ) ;
#37177=EDGE_CURVE ( 'NONE', #60489, #78013, #83826, .T. ) ;
#37216=ORIENTED_EDGE ( 'NONE', *, *, #20271, .F. ) ;
#37252=CARTESIAN_POINT ( 'NONE',  ( -147.0026986695708047, -210.7421749798627673, -21.50000000000000000 ) ) ;
#37291=EDGE_CURVE ( 'NONE', #54318, #60845, #29283, .T. ) ;
#37293=ORIENTED_EDGE ( 'NONE', *, *, #61083, .T. ) ;
#37355=LINE ( 'NONE', #66262, #53398 ) ;
#37368=CARTESIAN_POINT ( 'NONE',  ( 60.30377782462292657, -249.1633071459562530, -21.50000000000000000 ) ) ;
#37403=ORIENTED_EDGE ( 'NONE', *, *, #34428, .F. ) ;
#37424=EDGE_CURVE ( 'NONE', #60290, #22436, #86161, .T. ) ;
#37428=VERTEX_POINT ( 'NONE', #9 ) ;
#37463=VERTEX_POINT ( 'NONE', #71048 ) ;
#37491=TOROIDAL_SURFACE ( 'NONE', #38974, 160.1282194813176716, 1.000000000000000000 ) ;
#37560=EDGE_CURVE ( 'NONE', #43675, #40890, #45948, .T. ) ;
#37610=EDGE_LOOP ( 'NONE', ( #65047, #57827, #92251 ) ) ;
#37611=DIRECTION ( 'NONE',  ( 1.000000000000000000, 0.000000000000000000, 0.000000000000000000 ) ) ;
#37627=AXIS2_PLACEMENT_3D ( 'NONE', #32376, #11042, #76401 ) ;
#37686=AXIS2_PLACEMENT_3D ( 'NONE', #48555, #48086, #62815 ) ;
#37719=DIRECTION ( 'NONE',  ( 0.000000000000000000, 0.000000000000000000, -1.000000000000000000 ) ) ;
#37756=DIRECTION ( 'NONE',  ( -0.000000000000000000, -0.000000000000000000, 1.000000000000000000 ) ) ;
#37759=CONICAL_SURFACE ( 'NONE', #90657, 5.024999999999987921, 0.7853981633974482790 ) ;
#37793=VERTEX_POINT ( 'NONE', #88011 ) ;
#37794=CYLINDRICAL_SURFACE ( 'NONE', #85147, 7.500000000000012434 ) ;
#37797=EDGE_CURVE ( 'NONE', #87117, #58726, #6652, .T. ) ;
#37809=DIRECTION ( 'NONE',  ( 0.8946341770721968345, 0.4467993836324679613, 0.000000000000000000 ) ) ;
#37821=DIRECTION ( 'NONE',  ( 1.000000000000000000, 0.000000000000000000, 0.000000000000000000 ) ) ;
#37845=ORIENTED_EDGE ( 'NONE', *, *, #59688, .T. ) ;
#37853=EDGE_CURVE ( 'NONE', #16441, #90518, #67209, .T. ) ;
#37863=CARTESIAN_POINT ( 'NONE',  ( 188.7149167944524493, -12.49482340714361506, 10.00000000000000000 ) ) ;
#37867=CARTESIAN_POINT ( 'NONE',  ( 73.43068321062709458, -134.2391364535880598, 0.000000000000000000 ) ) ;
#37911=CARTESIAN_POINT ( 'NONE',  ( -23.68628624284178130, -43.55766379199612004, 22.50000000000000000 ) ) ;
#37945=CARTESIAN_POINT ( 'NONE',  ( 123.4306832106270946, -134.2391364535880882, 4.999999999999990230 ) ) ;
#37979=ORIENTED_EDGE ( 'NONE', *, *, #4151, .T. ) ;
#38033=CARTESIAN_POINT ( 'NONE',  ( 17.06571399127465583, -89.54582641780471874, 21.50000000000000000 ) ) ;
#38034=EDGE_CURVE ( 'NONE', #74706, #29017, #17244, .T. ) ;
#38062=ORIENTED_EDGE ( 'NONE', *, *, #56630, .F. ) ;
#38149=AXIS2_PLACEMENT_3D ( 'NONE', #75129, #54267, #24936 ) ;
#38183=CARTESIAN_POINT ( 'NONE',  ( -23.68628624284178130, -43.55766379199612004, -21.50000000000000000 ) ) ;
#38224=CIRCLE ( 'NONE', #68456, 7.999999999999992895 ) ;
#38247=LINE ( 'NONE', #60992, #1962 ) ;
#38265=EDGE_CURVE ( 'NONE', #72058, #29328, #9888, .T. ) ;
#38279=CARTESIAN_POINT ( 'NONE',  ( 125.0516381006427338, 8.053287430127817004, -21.50000000000000000 ) ) ;
#38290=AXIS2_PLACEMENT_3D ( 'NONE', #30731, #74753, #8477 ) ;
#38292=CARTESIAN_POINT ( 'NONE',  ( -18.20453976106250948, -63.49190233628851132, -21.50000000000000000 ) ) ;
#38295=TOROIDAL_SURFACE ( 'NONE', #35274, 2.000000000000000000, 1.000000000000000000 ) ;
#38355=ORIENTED_EDGE ( 'NONE', *, *, #90249, .F. ) ;
#38369=AXIS2_PLACEMENT_3D ( 'NONE', #87095, #49259, #85239 ) ;
#38426=CIRCLE ( 'NONE', #61107, 15.36528803885689420 ) ;
#38462=EDGE_CURVE ( 'NONE', #33292, #55168, #70178, .T. ) ;
#38502=ORIENTED_EDGE ( 'NONE', *, *, #18406, .F. ) ;
#38515=EDGE_CURVE ( 'NONE', #9328, #83649, #36914, .T. ) ;
#38650=DIRECTION ( 'NONE',  ( -1.000000000000000000, 0.000000000000000000, 0.000000000000000000 ) ) ;
#38784=FACE_OUTER_BOUND ( 'NONE', #80838, .T. ) ;
#38799=ADVANCED_FACE ( 'NONE', ( #48191 ), #41556, .T. ) ;
#38837=ORIENTED_EDGE ( 'NONE', *, *, #58308, .T. ) ;
#38852=EDGE_CURVE ( 'NONE', #30831, #783, #18722, .T. ) ;
#38885=DIRECTION ( 'NONE',  ( -0.000000000000000000, 1.000000000000000000, -0.000000000000000000 ) ) ;
#38973=DIRECTION ( 'NONE',  ( -0.000000000000000000, -0.000000000000000000, 1.000000000000000000 ) ) ;
#38974=AXIS2_PLACEMENT_3D ( 'NONE', #23321, #81524, #9558 ) ;
#38977=DIRECTION ( 'NONE',  ( -0.000000000000000000, 1.000000000000000000, -0.000000000000000000 ) ) ;
#39023=ADVANCED_FACE ( 'NONE', ( #4193 ), #61128, .T. ) ;
#39053=ORIENTED_EDGE ( 'NONE', *, *, #27120, .F. ) ;
#39078=FACE_OUTER_BOUND ( 'NONE', #23820, .T. ) ;
#39086=DIRECTION ( 'NONE',  ( 1.000000000000000000, 0.000000000000000000, 0.000000000000000000 ) ) ;
#39104=DIRECTION ( 'NONE',  ( 1.000000000000000000, 0.000000000000000000, 0.000000000000000000 ) ) ;
#39136=EDGE_LOOP ( 'NONE', ( #61477, #74306, #29666, #91451 ) ) ;
#39228=EDGE_CURVE ( 'NONE', #6380, #57488, #57658, .T. ) ;
#39244=ORIENTED_EDGE ( 'NONE', *, *, #38852, .F. ) ;
#39249=ADVANCED_FACE ( 'NONE', ( #22134 ), #35416, .F. ) ;
#39272=ORIENTED_EDGE ( 'NONE', *, *, #9884, .T. ) ;
#39290=ORIENTED_EDGE ( 'NONE', *, *, #12262, .F. ) ;
#39296=CONICAL_SURFACE ( 'NONE', #16616, 4.999999999999990230, 1.029744258676648538 ) ;
#39321=DIRECTION ( 'NONE',  ( -0.000000000000000000, -1.000000000000000000, -0.000000000000000000 ) ) ;
#39323=CYLINDRICAL_SURFACE ( 'NONE', #68619, 1.000000000000000888 ) ;
#39325=CARTESIAN_POINT ( 'NONE',  ( 73.43068321062709458, -134.2391364535880598, 5.025000000000002132 ) ) ;
#39352=EDGE_CURVE ( 'NONE', #40992, #29264, #71882, .T. ) ;
#39353=CARTESIAN_POINT ( 'NONE',  ( 195.5881128153457098, 0.000000000000000000, 21.50000000000000000 ) ) ;
#39354=CIRCLE ( 'NONE', #74128, 203.9779373800640485 ) ;
#39392=CARTESIAN_POINT ( 'NONE',  ( 161.2494399300530290, -11.64849832608277325, -3.999999999999998224 ) ) ;
#39421=CARTESIAN_POINT ( 'NONE',  ( 73.43068321062709458, -134.2641364535880939, 0.000000000000000000 ) ) ;
#39431=CARTESIAN_POINT ( 'NONE',  ( 61.37083282337847123, -250.8548725835408391, -21.50000000000000000 ) ) ;
#39510=ORIENTED_EDGE ( 'NONE', *, *, #62017, .T. ) ;
#39545=DIRECTION ( 'NONE',  ( -0.000000000000000000, 1.000000000000000000, -0.000000000000000000 ) ) ;
#39593=ORIENTED_EDGE ( 'NONE', *, *, #47455, .T. ) ;
#39604=CARTESIAN_POINT ( 'NONE',  ( 222.8344101925596306, -44.55766379199611293, 22.08578643762690419 ) ) ;
#39628=DIRECTION ( 'NONE',  ( -0.000000000000000000, -0.000000000000000000, -1.000000000000000000 ) ) ;
#39639=VECTOR ( 'NONE', #45039, 1000.000000000000000 ) ;
#39658=DIRECTION ( 'NONE',  ( -0.000000000000000000, 0.000000000000000000, -1.000000000000000000 ) ) ;
#39660=( BOUNDED_CURVE ( )  B_SPLINE_CURVE ( 3, ( #41678, #92336, #6667, #56389 ),
 .UNSPECIFIED., .F., .F. ) 
 B_SPLINE_CURVE_WITH_KNOTS ( ( 4, 4 ),
 ( 3.141592653589779349, 4.712388980384689674 ),
 .UNSPECIFIED. ) 
 CURVE ( )  GEOMETRIC_REPRESENTATION_ITEM ( )  RATIONAL_B_SPLINE_CURVE ( ( 1.000000000000000000, 0.8047378541243617178, 0.8047378541243617178, 1.000000000000000000 ) ) 
 REPRESENTATION_ITEM ( '' )  );
#39690=AXIS2_PLACEMENT_3D ( 'NONE', #84388, #47937, #63131 ) ;
#39732=SHAPE_DEFINITION_REPRESENTATION ( #49709, #42162 ) ;
#39839=EDGE_LOOP ( 'NONE', ( #6016, #32768 ) ) ;
#39872=ORIENTED_EDGE ( 'NONE', *, *, #22475, .T. ) ;
#39926=ORIENTED_EDGE ( 'NONE', *, *, #22600, .F. ) ;
#39989=ORIENTED_EDGE ( 'NONE', *, *, #84897, .F. ) ;
#39990=AXIS2_PLACEMENT_3D ( 'NONE', #36985, #1458, #80522 ) ;
#40004=CIRCLE ( 'NONE', #12827, 160.1282194813176716 ) ;
#40023=CARTESIAN_POINT ( 'NONE',  ( 222.4306832106270804, -135.2391364535880882, 21.50000000000000000 ) ) ;
#40132=CARTESIAN_POINT ( 'NONE',  ( -35.09237171215954021, -122.5496321078137356, 21.50000000000000000 ) ) ;
#40133=CARTESIAN_POINT ( 'NONE',  ( 139.6925840978351516, 15.36528803885690664, -22.50000000000000000 ) ) ;
#40276=CARTESIAN_POINT ( 'NONE',  ( 143.6449502718966755, 5.787831549089307747E-16, 22.08578643762690064 ) ) ;
#40336=DIRECTION ( 'NONE',  ( 1.000000000000000000, 0.000000000000000000, 0.000000000000000000 ) ) ;
#40420=ORIENTED_EDGE ( 'NONE', *, *, #91737, .F. ) ;
#40423=EDGE_CURVE ( 'NONE', #55168, #33292, #65548, .T. ) ;
#40467=CIRCLE ( 'NONE', #51122, 1.000000000000000888 ) ;
#40475=DIRECTION ( 'NONE',  ( 0.000000000000000000, 0.000000000000000000, -1.000000000000000000 ) ) ;
#40493=FACE_OUTER_BOUND ( 'NONE', #80313, .T. ) ;
#40510=EDGE_CURVE ( 'NONE', #56465, #48629, #80814, .T. ) ;
#40530=DIRECTION ( 'NONE',  ( 0.000000000000000000, 0.000000000000000000, -1.000000000000000000 ) ) ;
#40534=EDGE_CURVE ( 'NONE', #26246, #60290, #68553, .T. ) ;
#40605=DIRECTION ( 'NONE',  ( -1.000000000000000000, 0.000000000000000000, 0.000000000000000000 ) ) ;
#40665=EDGE_CURVE ( 'NONE', #75656, #93680, #36437, .T. ) ;
#40715=AXIS2_PLACEMENT_3D ( 'NONE', #59394, #8709, #45610 ) ;
#40752=FACE_BOUND ( 'NONE', #56347, .T. ) ;
#40768=ORIENTED_EDGE ( 'NONE', *, *, #86200, .F. ) ;
#40773=DIRECTION ( 'NONE',  ( 0.000000000000000000, 0.000000000000000000, 1.000000000000000000 ) ) ;
#40879=DIRECTION ( 'NONE',  ( 1.000000000000000000, 0.000000000000000000, 0.000000000000000000 ) ) ;
#40887=EDGE_LOOP ( 'NONE', ( #55953, #30515, #41522 ) ) ;
#40890=VERTEX_POINT ( 'NONE', #35038 ) ;
#40992=VERTEX_POINT ( 'NONE', #22232 ) ;
#41016=ORIENTED_EDGE ( 'NONE', *, *, #82386, .F. ) ;
#41030=DIRECTION ( 'NONE',  ( 0.000000000000000000, 0.000000000000000000, 1.000000000000000000 ) ) ;
#41034=ORIENTED_EDGE ( 'NONE', *, *, #90146, .T. ) ;
#41070=CARTESIAN_POINT ( 'NONE',  ( 139.6925840978351516, 15.36528803885690664, 22.50000000000000000 ) ) ;
#41118=VERTEX_POINT ( 'NONE', #66715 ) ;
#41173=CARTESIAN_POINT ( 'NONE',  ( -35.09237171215954021, -122.5496321078137356, -21.49999999999998579 ) ) ;
#41189=CARTESIAN_POINT ( 'NONE',  ( 228.6245981097501101, -141.7221692137691775, -21.50000000000000000 ) ) ;
#41200=EDGE_CURVE ( 'NONE', #77986, #65497, #37355, .T. ) ;
#41220=DIRECTION ( 'NONE',  ( -1.124465274301078034E-16, -1.000000000000000000, 0.000000000000000000 ) ) ;
#41245=ORIENTED_EDGE ( 'NONE', *, *, #44575, .T. ) ;
#41271=CARTESIAN_POINT ( 'NONE',  ( 221.8344101925596306, -0.9999999999999991118, 22.50000000000000000 ) ) ;
#41282=CARTESIAN_POINT ( 'NONE',  ( -23.40286736638519471, -122.5496321078137356, 21.50000000000000000 ) ) ;
#41299=CARTESIAN_POINT ( 'NONE',  ( 222.4306832106270804, -134.2391364535880882, 21.50000000000000000 ) ) ;
#41300=CARTESIAN_POINT ( 'NONE',  ( -36.09237171215955442, -122.5496321078137356, 21.50000000000000000 ) ) ;
#41309=DIRECTION ( 'NONE',  ( 0.000000000000000000, -1.000000000000000000, -0.000000000000000000 ) ) ;
#41325=AXIS2_PLACEMENT_3D ( 'NONE', #72421, #35506, #50157 ) ;
#41328=DIRECTION ( 'NONE',  ( -0.000000000000000000, 1.000000000000000000, -0.000000000000000000 ) ) ;
#41345=AXIS2_PLACEMENT_3D ( 'NONE', #78615, #14235, #13759 ) ;
#41365=ORIENTED_EDGE ( 'NONE', *, *, #12942, .F. ) ;
#41404=VECTOR ( 'NONE', #79552, 1000.000000000000000 ) ;
#41476=ORIENTED_EDGE ( 'NONE', *, *, #27512, .F. ) ;
#41480=VECTOR ( 'NONE', #74954, 1000.000000000000114 ) ;
#41510=LINE ( 'NONE', #56215, #29577 ) ;
#41522=ORIENTED_EDGE ( 'NONE', *, *, #27345, .T. ) ;
#41523=ORIENTED_EDGE ( 'NONE', *, *, #8883, .T. ) ;
#41554=DIRECTION ( 'NONE',  ( -1.000000000000000000, 0.000000000000000000, 0.000000000000000000 ) ) ;
#41556=CYLINDRICAL_SURFACE ( 'NONE', #20294, 161.1282194813176716 ) ;
#41562=AXIS2_PLACEMENT_3D ( 'NONE', #18098, #68769, #17644 ) ;
#41565=FACE_OUTER_BOUND ( 'NONE', #67856, .T. ) ;
#41578=ORIENTED_EDGE ( 'NONE', *, *, #6798, .T. ) ;
#41581=CARTESIAN_POINT ( 'NONE',  ( -36.09237171215955442, -55.96374926131388605, -22.50000000000000000 ) ) ;
#41591=VERTEX_POINT ( 'NONE', #40132 ) ;
#41609=ORIENTED_EDGE ( 'NONE', *, *, #9644, .F. ) ;
#41617=ORIENTED_EDGE ( 'NONE', *, *, #90766, .T. ) ;
#41678=CARTESIAN_POINT ( 'NONE',  ( 222.8344101925596306, 0.000000000000000000, -21.49999999999998579 ) ) ;
#41708=CARTESIAN_POINT ( 'NONE',  ( 195.5881128153457098, -0.9999999999999991118, 22.50000000000000000 ) ) ;
#41728=ADVANCED_FACE ( 'NONE', ( #10796 ), #3716, .T. ) ;
#41863=VERTEX_POINT ( 'NONE', #83230 ) ;
#41869=EDGE_LOOP ( 'NONE', ( #10596, #54566, #56686, #62704 ) ) ;
#42046=CIRCLE ( 'NONE', #35245, 1.000000000000000888 ) ;
#42068=CYLINDRICAL_SURFACE ( 'NONE', #21875, 4.000000000000003553 ) ;
#42087=ORIENTED_EDGE ( 'NONE', *, *, #63349, .T. ) ;
#42088=CIRCLE ( 'NONE', #1281, 7.500000000000012434 ) ;
#42140=CARTESIAN_POINT ( 'NONE',  ( -55.80257052418233599, -229.5268262511776527, 22.47499999999998721 ) ) ;
#42155=CARTESIAN_POINT ( 'NONE',  ( 73.43068321062709458, -178.2391364535880882, 0.000000000000000000 ) ) ;
#42162=SHAPE_REPRESENTATION ( 'cast Iron C-Frame Chassis', ( #18940 ), #770 ) ;
#42187=EDGE_LOOP ( 'NONE', ( #20900, #24748, #48498, #78350 ) ) ;
#42244=EDGE_CURVE ( 'NONE', #92063, #61209, #56547, .T. ) ;
#42256=CARTESIAN_POINT ( 'NONE',  ( -23.40286736638519471, -135.2391364535880598, -22.50000000000000000 ) ) ;
#42274=ORIENTED_EDGE ( 'NONE', *, *, #84910, .F. ) ;
#42277=FACE_OUTER_BOUND ( 'NONE', #46060, .T. ) ;
#42298=DIRECTION ( 'NONE',  ( -0.000000000000000000, -0.000000000000000000, -1.000000000000000000 ) ) ;
#42386=CARTESIAN_POINT ( 'NONE',  ( 60.83730532400069535, -250.0090898647485176, -22.49999999999998579 ) ) ;
#42448=DIRECTION ( 'NONE',  ( 1.124465274301078281E-16, 1.000000000000000000, -0.000000000000000000 ) ) ;
#42478=DIRECTION ( 'NONE',  ( 0.5335274993777835428, -0.8457827187922967171, 0.000000000000000000 ) ) ;
#42514=ADVANCED_FACE ( 'NONE', ( #61613 ), #39323, .T. ) ;
#42533=DIRECTION ( 'NONE',  ( 1.000000000000000000, 0.000000000000000000, 0.000000000000000000 ) ) ;
#42543=FACE_OUTER_BOUND ( 'NONE', #49886, .T. ) ;
#42546=EDGE_LOOP ( 'NONE', ( #51648, #39510, #84338, #61742 ) ) ;
#42574=CIRCLE ( 'NONE', #281, 5.025000000000002132 ) ;
#42595=CARTESIAN_POINT ( 'NONE',  ( 222.4306832106270804, -141.7221692137691775, 21.50000000000000000 ) ) ;
#42630=DIRECTION ( 'NONE',  ( 0.000000000000000000, 0.000000000000000000, 1.000000000000000000 ) ) ;
#42646=DIRECTION ( 'NONE',  ( 0.000000000000000000, 1.000000000000000000, 0.000000000000000000 ) ) ;
#42675=CARTESIAN_POINT ( 'NONE',  ( -147.8070425842518034, -211.3363389866113664, 21.50000000000000000 ) ) ;
#42707=CIRCLE ( 'NONE', #75959, 154.4364916446740210 ) ;
#42791=EDGE_CURVE ( 'NONE', #70176, #74347, #54024, .T. ) ;
#42830=AXIS2_PLACEMENT_3D ( 'NONE', #13627, #13169, #42478 ) ;
#42839=CONICAL_SURFACE ( 'NONE', #26206, 5.025000000000002132, 0.7853981633971707232 ) ;
#42854=CIRCLE ( 'NONE', #56541, 1.000000000000000888 ) ;
#42906=AXIS2_PLACEMENT_3D ( 'NONE', #74615, #31531, #9744 ) ;
#42920=ORIENTED_EDGE ( 'NONE', *, *, #37853, .F. ) ;
#42926=CARTESIAN_POINT ( 'NONE',  ( 196.7510731661265595, -142.7221692137691775, -21.50000000000000000 ) ) ;
#43005=LINE ( 'NONE', #14140, #84734 ) ;
#43015=AXIS2_PLACEMENT_3D ( 'NONE', #80494, #20885, #86199 ) ;
#43032=DIRECTION ( 'NONE',  ( -1.000000000000000000, 0.000000000000000000, 0.000000000000000000 ) ) ;
#43035=VERTEX_POINT ( 'NONE', #51008 ) ;
#43069=AXIS2_PLACEMENT_3D ( 'NONE', #32683, #18942, #61569 ) ;
#43122=EDGE_CURVE ( 'NONE', #57485, #51305, #30845, .T. ) ;
#43225=ORIENTED_EDGE ( 'NONE', *, *, #79581, .F. ) ;
#43232=ADVANCED_FACE ( 'NONE', ( #71890 ), #83737, .T. ) ;
#43313=DIRECTION ( 'NONE',  ( -1.000000000000000000, 0.000000000000000000, 0.000000000000000000 ) ) ;
#43317=CARTESIAN_POINT ( 'NONE',  ( 222.8344101925596306, -44.55766379199612004, 22.50000000000000000 ) ) ;
#43389=DIRECTION ( 'NONE',  ( 0.000000000000000000, 1.000000000000000000, 0.000000000000000000 ) ) ;
#43397=LINE ( 'NONE', #28739, #92650 ) ;
#43420=FACE_BOUND ( 'NONE', #81899, .T. ) ;
#43491=ORIENTED_EDGE ( 'NONE', *, *, #37797, .F. ) ;
#43508=CARTESIAN_POINT ( 'NONE',  ( -147.8070425842518034, -211.3363389866113664, 22.50000000000000000 ) ) ;
#43588=CARTESIAN_POINT ( 'NONE',  ( 139.6925840978351516, -43.55766379199612004, 21.50000000000000000 ) ) ;
#43614=DIRECTION ( 'NONE',  ( -1.000000000000000000, 0.000000000000000000, 0.000000000000000000 ) ) ;
#43643=EDGE_CURVE ( 'NONE', #63355, #26085, #23988, .T. ) ;
#43660=CARTESIAN_POINT ( 'NONE',  ( -23.68628624284178130, -43.55766379199612004, -22.50000000000000000 ) ) ;
#43675=VERTEX_POINT ( 'NONE', #16889 ) ;
#43678=DIRECTION ( 'NONE',  ( 0.000000000000000000, 1.000000000000000000, 0.000000000000000000 ) ) ;
#43680=ORIENTED_EDGE ( 'NONE', *, *, #75213, .T. ) ;
#43751=EDGE_CURVE ( 'NONE', #78013, #29264, #570, .T. ) ;
#43755=DIRECTION ( 'NONE',  ( -0.000000000000000000, -0.000000000000000000, -1.000000000000000000 ) ) ;
#43782=CIRCLE ( 'NONE', #86165, 4.000000000000003553 ) ;
#43856=DIRECTION ( 'NONE',  ( 0.5335274993777835428, -0.8457827187922967171, 0.000000000000000000 ) ) ;
#44041=EDGE_CURVE ( 'NONE', #82488, #22426, #18763, .T. ) ;
#44062=ORIENTED_EDGE ( 'NONE', *, *, #10535, .F. ) ;
#44097=EDGE_CURVE ( 'NONE', #75708, #58726, #19683, .T. ) ;
#44113=LINE ( 'NONE', #1053, #50207 ) ;
#44190=ORIENTED_EDGE ( 'NONE', *, *, #5345, .T. ) ;
#44192=CIRCLE ( 'NONE', #69889, 1.000000000000000888 ) ;
#44309=CARTESIAN_POINT ( 'NONE',  ( 196.7510731661265595, -141.7221692137691775, -21.50000000000000000 ) ) ;
#44380=ORIENTED_EDGE ( 'NONE', *, *, #73898, .T. ) ;
#44381=CARTESIAN_POINT ( 'NONE',  ( 0.000000000000000000, 0.000000000000000000, 10.00000000000000000 ) ) ;
#44387=ADVANCED_FACE ( 'NONE', ( #30421 ), #37491, .T. ) ;
#44390=CIRCLE ( 'NONE', #26216, 204.9779373800640485 ) ;
#44394=ORIENTED_EDGE ( 'NONE', *, *, #6688, .F. ) ;
#44411=EDGE_LOOP ( 'NONE', ( #35252, #53760, #93464, #27538 ) ) ;
#44452=AXIS2_PLACEMENT_3D ( 'NONE', #22006, #88235, #30489 ) ;
#44457=DIRECTION ( 'NONE',  ( -0.000000000000000000, 1.000000000000000000, -0.000000000000000000 ) ) ;
#44496=ORIENTED_EDGE ( 'NONE', *, *, #26979, .T. ) ;
#44499=CARTESIAN_POINT ( 'NONE',  ( 194.5881128153457098, 0.000000000000000000, 21.50000000000000000 ) ) ;
#44511=DIRECTION ( 'NONE',  ( -0.000000000000000000, 1.000000000000000000, 0.000000000000000000 ) ) ;
#44512=ADVANCED_FACE ( 'NONE', ( #24714 ), #46469, .T. ) ;
#44526=VERTEX_POINT ( 'NONE', #63066 ) ;
#44570=ORIENTED_EDGE ( 'NONE', *, *, #1420, .F. ) ;
#44575=EDGE_CURVE ( 'NONE', #9328, #2619, #29947, .T. ) ;
#44602=DIRECTION ( 'NONE',  ( 0.000000000000000000, 0.000000000000000000, 1.000000000000000000 ) ) ;
#44610=CONICAL_SURFACE ( 'NONE', #77901, 5.025000000000002132, 0.7853981633971707232 ) ;
#44619=ADVANCED_FACE ( 'NONE', ( #40752, #76312, #5752, #61642 ), #62105, .F. ) ;
#44668=ORIENTED_EDGE ( 'NONE', *, *, #47032, .F. ) ;
#44672=VERTEX_POINT ( 'NONE', #41708 ) ;
#44714=ORIENTED_EDGE ( 'NONE', *, *, #26543, .T. ) ;
#44739=CARTESIAN_POINT ( 'NONE',  ( 200.9306832106271088, -134.2391364535880882, 0.000000000000000000 ) ) ;
#44781=DIRECTION ( 'NONE',  ( -0.000000000000000000, -0.000000000000000000, -1.000000000000000000 ) ) ;
#44862=LINE ( 'NONE', #66210, #82029 ) ;
#44867=VERTEX_POINT ( 'NONE', #27050 ) ;
#44894=FACE_OUTER_BOUND ( 'NONE', #7418, .T. ) ;
#44951=DIRECTION ( 'NONE',  ( -1.000000000000000000, 0.000000000000000000, 0.000000000000000000 ) ) ;
#44970=DIRECTION ( 'NONE',  ( -0.000000000000000000, 1.000000000000000000, -0.000000000000000000 ) ) ;
#45025=EDGE_CURVE ( 'NONE', #87746, #58890, #12373, .T. ) ;
#45039=DIRECTION ( 'NONE',  ( -1.000000000000000000, -0.000000000000000000, -0.000000000000000000 ) ) ;
#45084=ORIENTED_EDGE ( 'NONE', *, *, #56630, .T. ) ;
#45145=DIRECTION ( 'NONE',  ( -0.000000000000000000, -0.000000000000000000, -1.000000000000000000 ) ) ;
#45170=DIRECTION ( 'NONE',  ( -0.8457827187922972723, -0.5335274993777825436, -0.000000000000000000 ) ) ;
#45248=CONICAL_SURFACE ( 'NONE', #4453, 4.999999999999990230, 1.029744258676656754 ) ;
#45260=DIRECTION ( 'NONE',  ( -0.5941640067486159138, 0.8043439146810467122, 0.000000000000000000 ) ) ;
#45261=DIRECTION ( 'NONE',  ( -1.000000000000000000, 0.000000000000000000, 0.000000000000000000 ) ) ;
#45280=CARTESIAN_POINT ( 'NONE',  ( 194.7510731661265595, -164.3527196417747689, -21.50000000000000000 ) ) ;
#45328=EDGE_CURVE ( 'NONE', #20911, #15284, #35088, .T. ) ;
#45392=CYLINDRICAL_SURFACE ( 'NONE', #333, 1.000000000000000888 ) ;
#45415=ADVANCED_FACE ( 'NONE', ( #49760 ), #79593, .T. ) ;
#45445=ORIENTED_EDGE ( 'NONE', *, *, #87845, .T. ) ;
#45610=DIRECTION ( 'NONE',  ( 1.000000000000000000, 0.000000000000000000, 0.000000000000000000 ) ) ;
#45614=CARTESIAN_POINT ( 'NONE',  ( 61.37083282337847123, -250.8548725835408391, 22.50000000000000000 ) ) ;
#45632=DIRECTION ( 'NONE',  ( -0.000000000000000000, -0.000000000000000000, 1.000000000000000000 ) ) ;
#45711=FACE_OUTER_BOUND ( 'NONE', #25920, .T. ) ;
#45719=CIRCLE ( 'NONE', #53303, 4.000000000000003553 ) ;
#45734=EDGE_CURVE ( 'NONE', #29017, #41118, #80496, .T. ) ;
#45753=AXIS2_PLACEMENT_3D ( 'NONE', #19929, #84310, #19006 ) ;
#45765=ORIENTED_EDGE ( 'NONE', *, *, #80305, .T. ) ;
#45790=VECTOR ( 'NONE', #40336, 1000.000000000000000 ) ;
#45795=ORIENTED_EDGE ( 'NONE', *, *, #34350, .T. ) ;
#45803=AXIS2_PLACEMENT_3D ( 'NONE', #4906, #25283, #31920 ) ;
#45813=VECTOR ( 'NONE', #36780, 1000.000000000000000 ) ;
#45861=DIRECTION ( 'NONE',  ( -0.000000000000000000, -0.000000000000000000, -1.000000000000000000 ) ) ;
#45948=CIRCLE ( 'NONE', #89806, 204.9779373800640485 ) ;
#45995=AXIS2_PLACEMENT_3D ( 'NONE', #23848, #74501, #78145 ) ;
#46012=DIRECTION ( 'NONE',  ( -0.000000000000000000, 1.000000000000000000, -0.000000000000000000 ) ) ;
#46033=VERTEX_POINT ( 'NONE', #52545 ) ;
#46060=EDGE_LOOP ( 'NONE', ( #1463, #59820, #14056, #10365 ) ) ;
#46087=FACE_OUTER_BOUND ( 'NONE', #16809, .T. ) ;
#46090=TOROIDAL_SURFACE ( 'NONE', #11361, 154.4364916446740210, 1.000000000000000000 ) ;
#46147=ORIENTED_EDGE ( 'NONE', *, *, #82544, .T. ) ;
#46225=DIRECTION ( 'NONE',  ( -0.000000000000000000, 1.000000000000000000, 0.000000000000000000 ) ) ;
#46261=DIRECTION ( 'NONE',  ( 0.8457827187922972723, 0.5335274993777825436, 0.000000000000000000 ) ) ;
#46350=DIRECTION ( 'NONE',  ( 0.000000000000000000, 0.000000000000000000, -1.000000000000000000 ) ) ;
#46353=DIRECTION ( 'NONE',  ( -0.000000000000000000, -0.000000000000000000, 1.000000000000000000 ) ) ;
#46408=DIRECTION ( 'NONE',  ( 0.000000000000000000, 0.000000000000000000, 1.000000000000000000 ) ) ;
#46457=CARTESIAN_POINT ( 'NONE',  ( -23.68628624284178130, -43.55766379199612004, -21.50000000000000000 ) ) ;
#46469=CYLINDRICAL_SURFACE ( 'NONE', #17843, 1.000000000000000888 ) ;
#46495=FACE_OUTER_BOUND ( 'NONE', #3300, .T. ) ;
#46536=DIRECTION ( 'NONE',  ( -1.000000000000000000, -0.000000000000000000, -0.000000000000000000 ) ) ;
#46546=FACE_OUTER_BOUND ( 'NONE', #57060, .T. ) ;
#46556=DIRECTION ( 'NONE',  ( -1.000000000000000000, 0.000000000000000000, 0.000000000000000000 ) ) ;
#46725=ORIENTED_EDGE ( 'NONE', *, *, #33278, .T. ) ;
#46734=ORIENTED_EDGE ( 'NONE', *, *, #45734, .T. ) ;
#46744=VECTOR ( 'NONE', #74411, 1000.000000000000000 ) ;
#46808=CARTESIAN_POINT ( 'NONE',  ( 184.7149167944524493, -12.49482340714361506, 9.974999999999996092 ) ) ;
#46809=VECTOR ( 'NONE', #22924, 1000.000000000000000 ) ;
#46828=CARTESIAN_POINT ( 'NONE',  ( 73.43068321062709458, -134.2391364535880598, -5.025000000000002132 ) ) ;
#46850=CARTESIAN_POINT ( 'NONE',  ( 60.83730532400070246, -250.0090898647485176, 21.50000000000000000 ) ) ;
#46866=VERTEX_POINT ( 'NONE', #33885 ) ;
#46897=DIRECTION ( 'NONE',  ( 0.000000000000000000, 1.000000000000000000, 0.000000000000000000 ) ) ;
#46910=EDGE_CURVE ( 'NONE', #25794, #13434, #67789, .T. ) ;
#46928=CARTESIAN_POINT ( 'NONE',  ( 123.4306832106270946, -178.2391364535880882, 0.000000000000000000 ) ) ;
#46933=CIRCLE ( 'NONE', #3096, 1.000000000000000888 ) ;
#46952=FACE_OUTER_BOUND ( 'NONE', #55962, .T. ) ;
#46977=VERTEX_POINT ( 'NONE', #4070 ) ;
#46994=FACE_OUTER_BOUND ( 'NONE', #10266, .T. ) ;
#47032=EDGE_CURVE ( 'NONE', #23241, #34073, #42088, .T. ) ;
#47085=AXIS2_PLACEMENT_3D ( 'NONE', #93161, #28314, #41554 ) ;
#47090=ORIENTED_EDGE ( 'NONE', *, *, #50938, .F. ) ;
#47173=ORIENTED_EDGE ( 'NONE', *, *, #26543, .F. ) ;
#47184=DIRECTION ( 'NONE',  ( -1.000000000000000000, 0.000000000000000000, 0.000000000000000000 ) ) ;
#47201=CARTESIAN_POINT ( 'NONE',  ( 194.5881128153457098, -26.00396092263537540, 10.00000000000000178 ) ) ;
#47207=CARTESIAN_POINT ( 'NONE',  ( 2.197429475817664013, -229.5268262511776527, -22.50000000000000000 ) ) ;
#47220=ORIENTED_EDGE ( 'NONE', *, *, #16696, .T. ) ;
#47248=DIRECTION ( 'NONE',  ( -0.000000000000000000, -0.000000000000000000, -1.000000000000000000 ) ) ;
#47280=ORIENTED_EDGE ( 'NONE', *, *, #68560, .F. ) ;
#47310=ORIENTED_EDGE ( 'NONE', *, *, #77831, .T. ) ;
#47330=AXIS2_PLACEMENT_3D ( 'NONE', #40133, #39658, #68581 ) ;
#47364=CARTESIAN_POINT ( 'NONE',  ( -36.09237171215956863, 15.36528803885690664, 21.50000000000000000 ) ) ;
#47382=ORIENTED_EDGE ( 'NONE', *, *, #14909, .T. ) ;
#47400=DIRECTION ( 'NONE',  ( 1.000000000000000000, 0.000000000000000000, 0.000000000000000000 ) ) ;
#47417=ORIENTED_EDGE ( 'NONE', *, *, #2712, .T. ) ;
#47419=EDGE_LOOP ( 'NONE', ( #2846, #51891, #36509, #75598 ) ) ;
#47429=EDGE_LOOP ( 'NONE', ( #81577, #86213, #42274, #69360, #23831, #78715, #89116, #77380 ) ) ;
#47451=ORIENTED_EDGE ( 'NONE', *, *, #12262, .T. ) ;
#47455=EDGE_CURVE ( 'NONE', #25970, #77341, #11883, .T. ) ;
#47464=LINE ( 'NONE', #5353, #70190 ) ;
#47518=AXIS2_PLACEMENT_3D ( 'NONE', #76071, #68037, #3163 ) ;
#47572=ORIENTED_EDGE ( 'NONE', *, *, #47032, .T. ) ;
#47665=CARTESIAN_POINT ( 'NONE',  ( 10.19742947581765691, -229.5268262511776527, -22.50000000000000000 ) ) ;
#47670=ORIENTED_EDGE ( 'NONE', *, *, #86916, .F. ) ;
#47731=DIRECTION ( 'NONE',  ( 1.000000000000000000, 0.000000000000000000, 0.000000000000000000 ) ) ;
#47737=DIRECTION ( 'NONE',  ( 0.000000000000000000, 0.000000000000000000, -1.000000000000000000 ) ) ;
#47751=DIRECTION ( 'NONE',  ( 0.000000000000000000, 0.000000000000000000, 1.000000000000000000 ) ) ;
#47761=ORIENTED_EDGE ( 'NONE', *, *, #44041, .T. ) ;
#47859=DIRECTION ( 'NONE',  ( -0.000000000000000000, 0.000000000000000000, 1.000000000000000000 ) ) ;
#47889=ORIENTED_EDGE ( 'NONE', *, *, #77831, .F. ) ;
#47937=DIRECTION ( 'NONE',  ( 0.000000000000000000, 1.000000000000000000, 0.000000000000000000 ) ) ;
#48032=ORIENTED_EDGE ( 'NONE', *, *, #87216, .T. ) ;
#48034=ADVANCED_FACE ( 'NONE', ( #2096 ), #30987, .F. ) ;
#48086=DIRECTION ( 'NONE',  ( -0.000000000000000000, -0.000000000000000000, 1.000000000000000000 ) ) ;
#48140=EDGE_LOOP ( 'NONE', ( #71186, #91570, #27393 ) ) ;
#48158=EDGE_CURVE ( 'NONE', #41591, #4350, #69405, .T. ) ;
#48191=FACE_OUTER_BOUND ( 'NONE', #65993, .T. ) ;
#48216=ADVANCED_FACE ( 'NONE', ( #84410 ), #62192, .F. ) ;
#48238=CARTESIAN_POINT ( 'NONE',  ( 165.2494399300530290, -11.64849832608277325, 10.00000000000000000 ) ) ;
#48275=ORIENTED_EDGE ( 'NONE', *, *, #67622, .T. ) ;
#48327=CARTESIAN_POINT ( 'NONE',  ( 143.6449502718966755, 0.000000000000000000, 21.50000000000000000 ) ) ;
#48364=TOROIDAL_SURFACE ( 'NONE', #90651, 203.9779373800640485, 1.000000000000000000 ) ;
#48439=ORIENTED_EDGE ( 'NONE', *, *, #38852, .T. ) ;
#48494=ADVANCED_FACE ( 'NONE', ( #83009 ), #84876, .T. ) ;
#48498=ORIENTED_EDGE ( 'NONE', *, *, #87845, .F. ) ;
#48555=CARTESIAN_POINT ( 'NONE',  ( 165.2494399300530290, -11.64849832608277325, 10.00000000000000000 ) ) ;
#48586=EDGE_LOOP ( 'NONE', ( #65566, #9240, #24506, #9137 ) ) ;
#48616=LINE ( 'NONE', #5564, #65824 ) ;
#48629=VERTEX_POINT ( 'NONE', #7228 ) ;
#48630=ORIENTED_EDGE ( 'NONE', *, *, #14407, .F. ) ;
#48664=DIRECTION ( 'NONE',  ( -1.000000000000000000, 0.000000000000000000, 0.000000000000000000 ) ) ;
#48693=EDGE_CURVE ( 'NONE', #37428, #60407, #25532, .T. ) ;
#48702=ORIENTED_EDGE ( 'NONE', *, *, #16793, .F. ) ;
#48715=VECTOR ( 'NONE', #55205, 1000.000000000000000 ) ;
#48770=DIRECTION ( 'NONE',  ( 0.000000000000000000, 0.000000000000000000, 1.000000000000000000 ) ) ;
#48804=CIRCLE ( 'NONE', #18609, 0.9999999999999896749 ) ;
#48813=EDGE_CURVE ( 'NONE', #8064, #90187, #71642, .T. ) ;
#48831=CIRCLE ( 'NONE', #8021, 1.000000000000000888 ) ;
#48862=ORIENTED_EDGE ( 'NONE', *, *, #5103, .T. ) ;
#48882=CARTESIAN_POINT ( 'NONE',  ( 165.2494399300530290, -11.64849832608277325, 10.00000000000000000 ) ) ;
#48942=CARTESIAN_POINT ( 'NONE',  ( 73.43068321062709458, -134.2641364535880939, -4.999999999999990230 ) ) ;
#49096=CIRCLE ( 'NONE', #23409, 204.9779373800640485 ) ;
#49116=ORIENTED_EDGE ( 'NONE', *, *, #2076, .F. ) ;
#49232=ORIENTED_EDGE ( 'NONE', *, *, #30767, .T. ) ;
#49259=DIRECTION ( 'NONE',  ( 0.000000000000000000, -1.000000000000000000, 0.000000000000000000 ) ) ;
#49313=EDGE_LOOP ( 'NONE', ( #84002, #13725, #70050 ) ) ;
#49321=EDGE_CURVE ( 'NONE', #14651, #70449, #21907, .T. ) ;
#49329=DIRECTION ( 'NONE',  ( -1.000000000000000000, 0.000000000000000000, 0.000000000000000000 ) ) ;
#49436=ORIENTED_EDGE ( 'NONE', *, *, #40510, .F. ) ;
#49573=LINE ( 'NONE', #11718, #32169 ) ;
#49593=CARTESIAN_POINT ( 'NONE',  ( 143.6449502718966755, -26.00396092263537540, 10.00000000000000178 ) ) ;
#49618=DIRECTION ( 'NONE',  ( 0.000000000000000000, -0.000000000000000000, 1.000000000000000000 ) ) ;
#49657=DIRECTION ( 'NONE',  ( -0.000000000000000000, -0.000000000000000000, 1.000000000000000000 ) ) ;
#49676=VECTOR ( 'NONE', #31258, 1000.000000000000000 ) ;
#49709=PRODUCT_DEFINITION_SHAPE ( 'NONE', 'NONE',  #12282 ) ;
#49728=CARTESIAN_POINT ( 'NONE',  ( -23.40286736638519471, -135.2391364535880598, 22.50000000000000000 ) ) ;
#49760=FACE_OUTER_BOUND ( 'NONE', #63339, .T. ) ;
#49853=EDGE_LOOP ( 'NONE', ( #7994, #31952, #51960, #5686, #77704, #86802, #853, #66700, #53512, #41617, #53975, #86951, #61626, #88215, #35671, #79612, #46147, #22169, #70084, #92499, #23692, #39272 ) ) ;
#49886=EDGE_LOOP ( 'NONE', ( #59960, #15309, #74479, #41476 ) ) ;
#50022=CARTESIAN_POINT ( 'NONE',  ( 184.7149167944524493, -12.49482340714361506, 10.00000000000000000 ) ) ;
#50034=CARTESIAN_POINT ( 'NONE',  ( -23.68628624284178130, -55.96374926131388605, 21.50000000000000000 ) ) ;
#50071=AXIS2_PLACEMENT_3D ( 'NONE', #14387, #15763, #73525 ) ;
#50094=DIRECTION ( 'NONE',  ( -0.000000000000000000, -0.000000000000000000, -1.000000000000000000 ) ) ;
#50121=EDGE_LOOP ( 'NONE', ( #21391, #77531, #25219, #44496 ) ) ;
#50155=ORIENTED_EDGE ( 'NONE', *, *, #80951, .F. ) ;
#50157=DIRECTION ( 'NONE',  ( 0.000000000000000000, 0.000000000000000000, 1.000000000000000000 ) ) ;
#50174=DIRECTION ( 'NONE',  ( 0.000000000000000000, 0.000000000000000000, -1.000000000000000000 ) ) ;
#50207=VECTOR ( 'NONE', #65942, 1000.000000000000000 ) ;
#50283=AXIS2_PLACEMENT_3D ( 'NONE', #66129, #59010, #93124 ) ;
#50302=AXIS2_PLACEMENT_3D ( 'NONE', #12856, #83373, #54502 ) ;
#50363=EDGE_CURVE ( 'NONE', #29264, #78013, #13531, .T. ) ;
#50388=VERTEX_POINT ( 'NONE', #84539 ) ;
#50417=CARTESIAN_POINT ( 'NONE',  ( 123.4306832106270946, -134.2641364535880939, 0.000000000000000000 ) ) ;
#50496=ORIENTED_EDGE ( 'NONE', *, *, #70607, .T. ) ;
#50497=DIRECTION ( 'NONE',  ( 0.000000000000000000, 0.000000000000000000, 1.000000000000000000 ) ) ;
#50546=CARTESIAN_POINT ( 'NONE',  ( -47.80257052418233599, -229.5268262511776527, 22.50000000000000000 ) ) ;
#50557=CIRCLE ( 'NONE', #9720, 154.4364916446740210 ) ;
#50572=FACE_OUTER_BOUND ( 'NONE', #87584, .T. ) ;
#50575=CARTESIAN_POINT ( 'NONE',  ( -22.78264641048746597, -118.9815703160634541, 21.50000000000000000 ) ) ;
#50602=CARTESIAN_POINT ( 'NONE',  ( 139.6925840978351232, -135.2391364535880882, 21.50000000000000000 ) ) ;
#50656=LINE ( 'NONE', #29809, #57920 ) ;
#50712=ADVANCED_FACE ( 'NONE', ( #8616 ), #15270, .F. ) ;
#50780=CIRCLE ( 'NONE', #59856, 12.40608546931776957 ) ;
#50781=DIRECTION ( 'NONE',  ( 0.000000000000000000, 1.000000000000000000, 0.000000000000000000 ) ) ;
#50938=EDGE_CURVE ( 'NONE', #22426, #72058, #9067, .T. ) ;
#50967=CARTESIAN_POINT ( 'NONE',  ( 196.7510731661265595, -142.7221692137691775, 21.50000000000000000 ) ) ;
#50999=ADVANCED_FACE ( 'NONE', ( #30881 ), #69477, .F. ) ;
#51008=CARTESIAN_POINT ( 'NONE',  ( 194.7510731661265595, -164.3527196417747689, 22.50000000000000000 ) ) ;
#51011=FACE_OUTER_BOUND ( 'NONE', #82042, .T. ) ;
#51025=DIRECTION ( 'NONE',  ( 0.000000000000000000, 0.000000000000000000, 1.000000000000000000 ) ) ;
#51084=ORIENTED_EDGE ( 'NONE', *, *, #57774, .T. ) ;
#51122=AXIS2_PLACEMENT_3D ( 'NONE', #88988, #65874, #88055 ) ;
#51127=EDGE_CURVE ( 'NONE', #13434, #32648, #24111, .T. ) ;
#51144=DIRECTION ( 'NONE',  ( -0.000000000000000000, -0.000000000000000000, -1.000000000000000000 ) ) ;
#51181=CARTESIAN_POINT ( 'NONE',  ( -23.68628624284178130, -44.55766379199612004, -21.49999999999998579 ) ) ;
#51305=VERTEX_POINT ( 'NONE', #3378 ) ;
#51353=AXIS2_PLACEMENT_3D ( 'NONE', #50417, #79322, #20138 ) ;
#51355=CARTESIAN_POINT ( 'NONE',  ( -39.58036566374939724, -229.5268262511776527, 21.50000000000000000 ) ) ;
#51419=DIRECTION ( 'NONE',  ( 0.000000000000000000, 0.000000000000000000, -1.000000000000000000 ) ) ;
#51429=EDGE_CURVE ( 'NONE', #18590, #93421, #4511, .T. ) ;
#51453=DIRECTION ( 'NONE',  ( 8.659560562354932858E-17, 0.7071067811865474617, -0.7071067811865474617 ) ) ;
#51481=DIRECTION ( 'NONE',  ( -0.000000000000000000, -0.000000000000000000, -1.000000000000000000 ) ) ;
#51544=ADVANCED_FACE ( 'NONE', ( #5278 ), #39296, .F. ) ;
#51550=TOROIDAL_SURFACE ( 'NONE', #28931, 8.222204860432942297, 1.000000000000000000 ) ;
#51636=CARTESIAN_POINT ( 'NONE',  ( 222.4306832106270804, -141.7221692137691775, -22.50000000000000000 ) ) ;
#51648=ORIENTED_EDGE ( 'NONE', *, *, #8814, .F. ) ;
#51672=DIRECTION ( 'NONE',  ( -1.000000000000000000, 0.000000000000000000, -0.000000000000000000 ) ) ;
#51697=VERTEX_POINT ( 'NONE', #27506 ) ;
#51716=CYLINDRICAL_SURFACE ( 'NONE', #50071, 4.000000000000003553 ) ;
#51756=EDGE_CURVE ( 'NONE', #15284, #3498, #31760, .T. ) ;
#51765=ORIENTED_EDGE ( 'NONE', *, *, #6503, .T. ) ;
#51785=DIRECTION ( 'NONE',  ( -0.000000000000000000, -0.000000000000000000, 1.000000000000000000 ) ) ;
#51816=CARTESIAN_POINT ( 'NONE',  ( -39.58036566374939724, -229.5268262511776527, 22.50000000000000000 ) ) ;
#51887=CIRCLE ( 'NONE', #62463, 12.68950434577434372 ) ;
#51891=ORIENTED_EDGE ( 'NONE', *, *, #88395, .F. ) ;
#51915=( NAMED_UNIT ( * ) PLANE_ANGLE_UNIT ( ) SI_UNIT ( $, .RADIAN. ) );
#51946=ORIENTED_EDGE ( 'NONE', *, *, #30285, .T. ) ;
#51960=ORIENTED_EDGE ( 'NONE', *, *, #71269, .T. ) ;
#51967=ADVANCED_FACE ( 'NONE', ( #57799 ), #86185, .F. ) ;
#52008=CARTESIAN_POINT ( 'NONE',  ( 139.6925840978351516, -0.9999999999999991118, 21.50000000000000000 ) ) ;
#52013=ORIENTED_EDGE ( 'NONE', *, *, #37424, .F. ) ;
#52032=LINE ( 'NONE', #16518, #12558 ) ;
#52071=EDGE_LOOP ( 'NONE', ( #41034, #30918, #83467 ) ) ;
#52128=ORIENTED_EDGE ( 'NONE', *, *, #76268, .F. ) ;
#52191=CARTESIAN_POINT ( 'NONE',  ( 139.6925840978351516, 0.000000000000000000, 22.50000000000000000 ) ) ;
#52208=ORIENTED_EDGE ( 'NONE', *, *, #57188, .F. ) ;
#52221=ORIENTED_EDGE ( 'NONE', *, *, #24174, .F. ) ;
#52258=CIRCLE ( 'NONE', #91589, 1.000000000000000888 ) ;
#52272=CARTESIAN_POINT ( 'NONE',  ( -47.80257052418233599, -229.5268262511776527, 22.50000000000000000 ) ) ;
#52294=ADVANCED_FACE ( 'NONE', ( #29844 ), #28731, .T. ) ;
#52334=LINE ( 'NONE', #293, #89808 ) ;
#52406=DIRECTION ( 'NONE',  ( 0.000000000000000000, -1.000000000000000000, 0.000000000000000000 ) ) ;
#52464=CARTESIAN_POINT ( 'NONE',  ( -35.09237171215954731, -55.96374926131387895, -21.50000000000000000 ) ) ;
#52545=CARTESIAN_POINT ( 'NONE',  ( 208.4306832106271088, -44.55766379199612004, 7.500000000000012434 ) ) ;
#52695=ORIENTED_EDGE ( 'NONE', *, *, #9884, .F. ) ;
#52721=CARTESIAN_POINT ( 'NONE',  ( -23.40286736638519471, -122.5496321078137356, 22.50000000000000000 ) ) ;
#52742=ORIENTED_EDGE ( 'NONE', *, *, #34428, .T. ) ;
#52806=ORIENTED_EDGE ( 'NONE', *, *, #37560, .T. ) ;
#52836=CARTESIAN_POINT ( 'NONE',  ( 161.2494399300530290, -11.64849832608277325, -3.999999999999998224 ) ) ;
#52845=( NAMED_UNIT ( * ) SI_UNIT ( $, .STERADIAN. ) SOLID_ANGLE_UNIT ( ) );
#52851=CARTESIAN_POINT ( 'NONE',  ( 125.9462722777150958, 8.500086813760361792, 21.50000000000000000 ) ) ;
#52864=FACE_OUTER_BOUND ( 'NONE', #42187, .T. ) ;
#52889=ORIENTED_EDGE ( 'NONE', *, *, #50363, .F. ) ;
#52902=CARTESIAN_POINT ( 'NONE',  ( 223.4306832106271372, -147.4436952405746695, -21.50000000000000000 ) ) ;
#52932=ADVANCED_FACE ( 'NONE', ( #38784 ), #48364, .T. ) ;
#52998=CARTESIAN_POINT ( 'NONE',  ( 195.0023263777187879, -0.4142135623730946459, 22.50000000000000000 ) ) ;
#53021=ORIENTED_EDGE ( 'NONE', *, *, #45025, .T. ) ;
#53026=EDGE_CURVE ( 'NONE', #76418, #25970, #89182, .T. ) ;
#53072=CARTESIAN_POINT ( 'NONE',  ( 208.4306832106270804, -324.2391364535881735, 0.000000000000000000 ) ) ;
#53093=EDGE_LOOP ( 'NONE', ( #37403, #80967, #18124, #33015 ) ) ;
#53131=ORIENTED_EDGE ( 'NONE', *, *, #2228, .F. ) ;
#53215=DIRECTION ( 'NONE',  ( 0.000000000000000000, 0.000000000000000000, 1.000000000000000000 ) ) ;
#53252=ORIENTED_EDGE ( 'NONE', *, *, #16816, .F. ) ;
#53259=EDGE_CURVE ( 'NONE', #3537, #10408, #30274, .T. ) ;
#53303=AXIS2_PLACEMENT_3D ( 'NONE', #59518, #10219, #39086 ) ;
#53314=LINE ( 'NONE', #31096, #17027 ) ;
#53363=CIRCLE ( 'NONE', #38290, 8.000000000000000000 ) ;
#53370=AXIS2_PLACEMENT_3D ( 'NONE', #76390, #38973, #83942 ) ;
#53393=LINE ( 'NONE', #69474, #74908 ) ;
#53398=VECTOR ( 'NONE', #44457, 1000.000000000000000 ) ;
#53470=AXIS2_PLACEMENT_3D ( 'NONE', #30169, #7011, #57667 ) ;
#53473=FACE_OUTER_BOUND ( 'NONE', #42546, .T. ) ;
#53512=ORIENTED_EDGE ( 'NONE', *, *, #48813, .T. ) ;
#53551=AXIS2_PLACEMENT_3D ( 'NONE', #83866, #47400, #91894 ) ;
#53587=ADVANCED_FACE ( 'NONE', ( #21222 ), #72658, .T. ) ;
#53597=AXIS2_PLACEMENT_3D ( 'NONE', #33716, #62628, #92396 ) ;
#53601=CARTESIAN_POINT ( 'NONE',  ( -35.09237171215954731, -55.96374926131388605, 21.50000000000000000 ) ) ;
#53626=CARTESIAN_POINT ( 'NONE',  ( 222.8344101925596306, -44.55766379199612004, 21.50000000000000000 ) ) ;
#53673=AXIS2_PLACEMENT_3D ( 'NONE', #89415, #10822, #67222 ) ;
#53722=EDGE_CURVE ( 'NONE', #90108, #9328, #43005, .T. ) ;
#53740=ORIENTED_EDGE ( 'NONE', *, *, #13993, .T. ) ;
#53755=ORIENTED_EDGE ( 'NONE', *, *, #14909, .F. ) ;
#53760=ORIENTED_EDGE ( 'NONE', *, *, #19908, .F. ) ;
#53813=DIRECTION ( 'NONE',  ( -0.000000000000000000, -0.000000000000000000, -1.000000000000000000 ) ) ;
#53886=ADVANCED_FACE ( 'NONE', ( #59551, #1304, #50572 ), #59074, .T. ) ;
#53965=ORIENTED_EDGE ( 'NONE', *, *, #70607, .F. ) ;
#53975=ORIENTED_EDGE ( 'NONE', *, *, #12686, .T. ) ;
#54005=EDGE_CURVE ( 'NONE', #70302, #51305, #87696, .T. ) ;
#54024=LINE ( 'NONE', #84296, #26299 ) ;
#54027=DIRECTION ( 'NONE',  ( 0.000000000000000000, 1.000000000000000000, 0.000000000000000000 ) ) ;
#54054=DIRECTION ( 'NONE',  ( -1.000000000000000000, 0.000000000000000000, 0.000000000000000000 ) ) ;
#54119=EDGE_CURVE ( 'NONE', #75846, #90412, #58160, .T. ) ;
#54137=ORIENTED_EDGE ( 'NONE', *, *, #34673, .F. ) ;
#54156=CYLINDRICAL_SURFACE ( 'NONE', #16754, 4.999999999999990230 ) ;
#54160=FACE_OUTER_BOUND ( 'NONE', #56942, .T. ) ;
#54267=DIRECTION ( 'NONE',  ( -0.000000000000000000, -0.000000000000000000, -1.000000000000000000 ) ) ;
#54294=ORIENTED_EDGE ( 'NONE', *, *, #83427, .F. ) ;
#54318=VERTEX_POINT ( 'NONE', #44739 ) ;
#54323=CYLINDRICAL_SURFACE ( 'NONE', #34096, 1.000000000000000888 ) ;
#54369=DIRECTION ( 'NONE',  ( -0.8946341770721975006, -0.4467993836324665180, 0.000000000000000000 ) ) ;
#54415=DIRECTION ( 'NONE',  ( -0.000000000000000000, -0.000000000000000000, -1.000000000000000000 ) ) ;
#54488=CARTESIAN_POINT ( 'NONE',  ( 161.2244399300530233, -11.64849832608277325, 10.00000000000000000 ) ) ;
#54498=ORIENTED_EDGE ( 'NONE', *, *, #53722, .F. ) ;
#54502=DIRECTION ( 'NONE',  ( 0.000000000000000000, 0.000000000000000000, -1.000000000000000000 ) ) ;
#54514=CARTESIAN_POINT ( 'NONE',  ( 223.4306832106270804, -134.2391364535880882, 22.50000000000000000 ) ) ;
#54537=CARTESIAN_POINT ( 'NONE',  ( 73.43068321062709458, -134.2391364535880598, 0.000000000000000000 ) ) ;
#54566=ORIENTED_EDGE ( 'NONE', *, *, #90249, .T. ) ;
#54618=CARTESIAN_POINT ( 'NONE',  ( 236.4625231464875128, -138.0407542764614846, 21.50000000000000000 ) ) ;
#54639=EDGE_CURVE ( 'NONE', #18590, #21234, #39354, .T. ) ;
#54642=EDGE_CURVE ( 'NONE', #41118, #46033, #67, .T. ) ;
#54719=AXIS2_PLACEMENT_3D ( 'NONE', #47364, #46897, #75798 ) ;
#54789=AXIS2_PLACEMENT_3D ( 'NONE', #39421, #88230, #23386 ) ;
#54790=DIRECTION ( 'NONE',  ( -1.000000000000000000, 0.000000000000000000, 0.000000000000000000 ) ) ;
#54791=AXIS2_PLACEMENT_3D ( 'NONE', #3148, #17373, #32030 ) ;
#54840=CARTESIAN_POINT ( 'NONE',  ( 195.7510731661265595, -143.7221692137691775, 21.50000000000000000 ) ) ;
#54854=DIRECTION ( 'NONE',  ( -0.000000000000000000, -0.000000000000000000, -1.000000000000000000 ) ) ;
#54957=LINE ( 'NONE', #83834, #30541 ) ;
#54978=CARTESIAN_POINT ( 'NONE',  ( -147.0026986695707762, -210.7421749798627388, 21.50000000000000000 ) ) ;
#54997=AXIS2_PLACEMENT_3D ( 'NONE', #50034, #56229, #57628 ) ;
#55057=DIRECTION ( 'NONE',  ( -0.000000000000000000, 1.000000000000000000, 0.000000000000000000 ) ) ;
#55076=AXIS2_PLACEMENT_3D ( 'NONE', #38033, #14899, #74037 ) ;
#55082=AXIS2_PLACEMENT_3D ( 'NONE', #76732, #90433, #48770 ) ;
#55139=ORIENTED_EDGE ( 'NONE', *, *, #51429, .F. ) ;
#55168=VERTEX_POINT ( 'NONE', #33808 ) ;
#55205=DIRECTION ( 'NONE',  ( 1.000000000000000000, -1.124465274301078034E-16, -0.000000000000000000 ) ) ;
#55220=CARTESIAN_POINT ( 'NONE',  ( 123.4306832106270946, -178.2391364535880882, 4.999999999999990230 ) ) ;
#55267=ORIENTED_EDGE ( 'NONE', *, *, #18425, .T. ) ;
#55292=DIRECTION ( 'NONE',  ( -1.000000000000000000, 0.000000000000000000, 0.000000000000000000 ) ) ;
#55311=PRODUCT_DEFINITION_FORMATION_WITH_SPECIFIED_SOURCE ( 'ANY', '', #73213, .NOT_KNOWN. ) ;
#55329=CARTESIAN_POINT ( 'NONE',  ( 195.7510731661265595, -143.7221692137691775, 22.50000000000000000 ) ) ;
#55365=DIRECTION ( 'NONE',  ( -0.000000000000000000, -0.000000000000000000, 1.000000000000000000 ) ) ;
#55372=LINE ( 'NONE', #46828, #64291 ) ;
#55409=VERTEX_POINT ( 'NONE', #48942 ) ;
#55430=EDGE_CURVE ( 'NONE', #70449, #70176, #74194, .T. ) ;
#55432=CARTESIAN_POINT ( 'NONE',  ( 222.4306832106270804, -134.2391364535880882, 22.50000000000000000 ) ) ;
#55459=DIRECTION ( 'NONE',  ( -1.000000000000000000, 0.000000000000000000, -0.000000000000000000 ) ) ;
#55502=ORIENTED_EDGE ( 'NONE', *, *, #92308, .F. ) ;
#55509=FACE_OUTER_BOUND ( 'NONE', #40887, .T. ) ;
#55547=ADVANCED_FACE ( 'NONE', ( #92018 ), #51550, .T. ) ;
#55702=AXIS2_PLACEMENT_3D ( 'NONE', #43588, #92845, #22285 ) ;
#55717=ORIENTED_EDGE ( 'NONE', *, *, #69834, .F. ) ;
#55731=ORIENTED_EDGE ( 'NONE', *, *, #63462, .F. ) ;
#55755=DIRECTION ( 'NONE',  ( -0.000000000000000000, -0.000000000000000000, -1.000000000000000000 ) ) ;
#55837=DIRECTION ( 'NONE',  ( -1.000000000000000000, 0.000000000000000000, 0.000000000000000000 ) ) ;
#55862=DIRECTION ( 'NONE',  ( 0.000000000000000000, 0.000000000000000000, -1.000000000000000000 ) ) ;
#55876=ORIENTED_EDGE ( 'NONE', *, *, #30492, .F. ) ;
#55912=DIRECTION ( 'NONE',  ( 0.000000000000000000, 0.000000000000000000, 1.000000000000000000 ) ) ;
#55924=DIRECTION ( 'NONE',  ( -0.000000000000000000, 1.000000000000000000, -0.000000000000000000 ) ) ;
#55926=FACE_OUTER_BOUND ( 'NONE', #21458, .T. ) ;
#55953=ORIENTED_EDGE ( 'NONE', *, *, #4532, .F. ) ;
#55962=EDGE_LOOP ( 'NONE', ( #14434, #31859, #25101, #92750 ) ) ;
#55999=LINE ( 'NONE', #61255, #56375 ) ;
#56040=FACE_BOUND ( 'NONE', #70723, .T. ) ;
#56104=EDGE_LOOP ( 'NONE', ( #36284, #79027, #60629, #43491 ) ) ;
#56106=PRODUCT_DEFINITION_CONTEXT ( 'detailed design', #84968, 'design' ) ;
#56200=ORIENTED_EDGE ( 'NONE', *, *, #8700, .F. ) ;
#56215=CARTESIAN_POINT ( 'NONE',  ( 222.8344101925596306, 0.000000000000000000, -21.50000000000000000 ) ) ;
#56229=DIRECTION ( 'NONE',  ( -0.000000000000000000, -0.000000000000000000, -1.000000000000000000 ) ) ;
#56248=AXIS2_PLACEMENT_3D ( 'NONE', #59043, #88373, #80342 ) ;
#56259=ADVANCED_FACE ( 'NONE', ( #59314 ), #51716, .F. ) ;
#56261=DIRECTION ( 'NONE',  ( -1.000000000000000000, 0.000000000000000000, 0.000000000000000000 ) ) ;
#56286=CYLINDRICAL_SURFACE ( 'NONE', #578, 11.40608546931776779 ) ;
#56302=ORIENTED_EDGE ( 'NONE', *, *, #12686, .F. ) ;
#56319=AXIS2_PLACEMENT_3D ( 'NONE', #84764, #56391, #62074 ) ;
#56347=EDGE_LOOP ( 'NONE', ( #89239, #25276 ) ) ;
#56365=DIRECTION ( 'NONE',  ( -0.000000000000000000, -1.000000000000000000, -0.000000000000000000 ) ) ;
#56375=VECTOR ( 'NONE', #62171, 1000.000000000000000 ) ;
#56389=CARTESIAN_POINT ( 'NONE',  ( 221.8344101925596306, -0.9999999999999997780, -22.50000000000000000 ) ) ;
#56391=DIRECTION ( 'NONE',  ( -0.000000000000000000, -0.000000000000000000, -1.000000000000000000 ) ) ;
#56418=FACE_OUTER_BOUND ( 'NONE', #84895, .T. ) ;
#56439=ADVANCED_FACE ( 'NONE', ( #74919 ), #81076, .T. ) ;
#56451=FACE_OUTER_BOUND ( 'NONE', #78324, .T. ) ;
#56465=VERTEX_POINT ( 'NONE', #53601 ) ;
#56487=EDGE_CURVE ( 'NONE', #14431, #90108, #31362, .T. ) ;
#56541=AXIS2_PLACEMENT_3D ( 'NONE', #41300, #20017, #27127 ) ;
#56547=CIRCLE ( 'NONE', #35373, 2.000000000000001776 ) ;
#56591=EDGE_LOOP ( 'NONE', ( #90569, #38837, #44570, #68411 ) ) ;
#56615=TOROIDAL_SURFACE ( 'NONE', #64203, 12.68950434577434372, 1.000000000000000000 ) ;
#56630=EDGE_CURVE ( 'NONE', #66913, #783, #81994, .T. ) ;
#56686=ORIENTED_EDGE ( 'NONE', *, *, #80835, .F. ) ;
#56709=CARTESIAN_POINT ( 'NONE',  ( 17.06571399127465583, -89.54582641780471874, 21.50000000000000000 ) ) ;
#56714=CARTESIAN_POINT ( 'NONE',  ( 222.4306832106270804, -147.4436952405746979, -22.50000000000000000 ) ) ;
#56742=VECTOR ( 'NONE', #43614, 1000.000000000000000 ) ;
#56773=DIRECTION ( 'NONE',  ( -1.000000000000000000, 0.000000000000000000, 0.000000000000000000 ) ) ;
#56790=ORIENTED_EDGE ( 'NONE', *, *, #40534, .F. ) ;
#56797=CARTESIAN_POINT ( 'NONE',  ( 222.4306832106270804, -141.7221692137691775, 22.50000000000000000 ) ) ;
#56800=ORIENTED_EDGE ( 'NONE', *, *, #27120, .T. ) ;
#56816=ORIENTED_EDGE ( 'NONE', *, *, #45734, .F. ) ;
#56942=EDGE_LOOP ( 'NONE', ( #31645, #993, #40768, #57917 ) ) ;
#57046=ADVANCED_FACE ( 'NONE', ( #57242 ), #91785, .F. ) ;
#57058=ORIENTED_EDGE ( 'NONE', *, *, #18534, .T. ) ;
#57060=EDGE_LOOP ( 'NONE', ( #4846, #35829, #83193, #204 ) ) ;
#57082=CARTESIAN_POINT ( 'NONE',  ( 222.4306832106270804, -142.7221692137691775, 21.50000000000000000 ) ) ;
#57143=CARTESIAN_POINT ( 'NONE',  ( -22.78264641048746597, -118.9815703160634541, -21.50000000000000000 ) ) ;
#57173=CARTESIAN_POINT ( 'NONE',  ( 123.4306832106270946, -134.2641364535880939, 0.000000000000000000 ) ) ;
#57188=EDGE_CURVE ( 'NONE', #30831, #90289, #79925, .T. ) ;
#57190=FACE_OUTER_BOUND ( 'NONE', #49853, .T. ) ;
#57216=DIRECTION ( 'NONE',  ( 0.000000000000000000, 1.000000000000000000, 0.000000000000000000 ) ) ;
#57242=FACE_OUTER_BOUND ( 'NONE', #88867, .T. ) ;
#57259=ORIENTED_EDGE ( 'NONE', *, *, #7154, .T. ) ;
#57485=VERTEX_POINT ( 'NONE', #74689 ) ;
#57488=VERTEX_POINT ( 'NONE', #2721 ) ;
#57536=CARTESIAN_POINT ( 'NONE',  ( 196.7510731661265595, -143.7221692137691775, 22.50000000000000000 ) ) ;
#57538=CIRCLE ( 'NONE', #9164, 1.000000000000000888 ) ;
#57623=CARTESIAN_POINT ( 'NONE',  ( 188.7149167944524493, -12.49482340714361506, 9.974999999999996092 ) ) ;
#57625=CARTESIAN_POINT ( 'NONE',  ( -47.80257052418233599, -229.5268262511776527, 22.50000000000000000 ) ) ;
#57628=DIRECTION ( 'NONE',  ( -1.000000000000000000, 0.000000000000000000, 0.000000000000000000 ) ) ;
#57658=LINE ( 'NONE', #20274, #85297 ) ;
#57664=VECTOR ( 'NONE', #59793, 1000.000000000000000 ) ;
#57667=DIRECTION ( 'NONE',  ( -1.000000000000000000, 0.000000000000000000, 0.000000000000000000 ) ) ;
#57701=DIRECTION ( 'NONE',  ( -0.000000000000000000, -0.000000000000000000, 1.000000000000000000 ) ) ;
#57722=ORIENTED_EDGE ( 'NONE', *, *, #34673, .T. ) ;
#57774=EDGE_CURVE ( 'NONE', #15223, #77294, #89386, .T. ) ;
#57785=DIRECTION ( 'NONE',  ( 0.000000000000000000, -1.000000000000000000, 0.000000000000000000 ) ) ;
#57799=FACE_OUTER_BOUND ( 'NONE', #26987, .T. ) ;
#57827=ORIENTED_EDGE ( 'NONE', *, *, #4015, .T. ) ;
#57841=LINE ( 'NONE', #59234, #56742 ) ;
#57893=CARTESIAN_POINT ( 'NONE',  ( 73.43068321062709458, -134.2641364535880939, 4.999999999999990230 ) ) ;
#57917=ORIENTED_EDGE ( 'NONE', *, *, #67180, .F. ) ;
#57920=VECTOR ( 'NONE', #72887, 1000.000000000000000 ) ;
#57934=VECTOR ( 'NONE', #54027, 1000.000000000000000 ) ;
#57938=VECTOR ( 'NONE', #62211, 1000.000000000000000 ) ;
#57949=AXIS2_PLACEMENT_3D ( 'NONE', #82282, #81803, #82738 ) ;
#58006=LINE ( 'NONE', #43317, #66517 ) ;
#58085=CARTESIAN_POINT ( 'NONE',  ( 125.9462722777150958, 8.500086813760361792, -21.49999999999998579 ) ) ;
#58090=CIRCLE ( 'NONE', #62623, 1.000000000000000888 ) ;
#58095=ADVANCED_FACE ( 'NONE', ( #61883 ), #76557, .T. ) ;
#58160=LINE ( 'NONE', #87005, #86220 ) ;
#58221=EDGE_LOOP ( 'NONE', ( #24290, #84005, #58222, #86071 ) ) ;
#58222=ORIENTED_EDGE ( 'NONE', *, *, #65538, .T. ) ;
#58242=AXIS2_PLACEMENT_3D ( 'NONE', #56797, #6592, #43032 ) ;
#58254=DIRECTION ( 'NONE',  ( 0.000000000000000000, 0.000000000000000000, 1.000000000000000000 ) ) ;
#58308=EDGE_CURVE ( 'NONE', #60290, #20083, #13866, .T. ) ;
#58433=EDGE_LOOP ( 'NONE', ( #70432, #16811, #6713, #47090 ) ) ;
#58441=EDGE_LOOP ( 'NONE', ( #34404, #71663 ) ) ;
#58554=DIRECTION ( 'NONE',  ( -1.000000000000000000, 0.000000000000000000, 0.000000000000000000 ) ) ;
#58616=DIRECTION ( 'NONE',  ( 0.000000000000000000, 0.000000000000000000, 1.000000000000000000 ) ) ;
#58642=VERTEX_POINT ( 'NONE', #42256 ) ;
#58726=VERTEX_POINT ( 'NONE', #70703 ) ;
#58890=VERTEX_POINT ( 'NONE', #66386 ) ;
#58941=ORIENTED_EDGE ( 'NONE', *, *, #19812, .T. ) ;
#58995=APPLICATION_CONTEXT ( 'automotive_design' ) ;
#59010=DIRECTION ( 'NONE',  ( 0.000000000000000000, 0.000000000000000000, 1.000000000000000000 ) ) ;
#59016=ORIENTED_EDGE ( 'NONE', *, *, #19908, .T. ) ;
#59017=DIRECTION ( 'NONE',  ( -0.8457827187922968282, -0.5335274993777835428, -5.868796551457945175E-15 ) ) ;
#59043=CARTESIAN_POINT ( 'NONE',  ( 123.4306832106270946, -134.2391364535880882, 0.000000000000000000 ) ) ;
#59045=EDGE_CURVE ( 'NONE', #71577, #6380, #44113, .T. ) ;
#59074=PLANE ( 'NONE',  #89247 ) ;
#59076=CARTESIAN_POINT ( 'NONE',  ( 60.83289261295102079, -250.0118895884541530, 21.50000000000000000 ) ) ;
#59104=EDGE_LOOP ( 'NONE', ( #77891, #21960, #75814, #15519 ) ) ;
#59234=CARTESIAN_POINT ( 'NONE',  ( 139.6925840978351516, 0.000000000000000000, -21.50000000000000000 ) ) ;
#59296=CARTESIAN_POINT ( 'NONE',  ( 222.4306832106270804, -135.2391364535880882, 21.50000000000000000 ) ) ;
#59314=FACE_OUTER_BOUND ( 'NONE', #16691, .T. ) ;
#59355=VERTEX_POINT ( 'NONE', #43660 ) ;
#59363=EDGE_LOOP ( 'NONE', ( #76100, #73071, #50496, #54137 ) ) ;
#59364=CARTESIAN_POINT ( 'NONE',  ( -47.80257052418233599, -229.5268262511776527, 21.50000000000000000 ) ) ;
#59394=CARTESIAN_POINT ( 'NONE',  ( 184.7149167944524493, -12.49482340714361506, -3.999999999999998224 ) ) ;
#59421=LINE ( 'NONE', #15865, #23683 ) ;
#59505=VECTOR ( 'NONE', #82669, 1000.000000000000000 ) ;
#59508=DIRECTION ( 'NONE',  ( -0.000000000000000000, -0.000000000000000000, 1.000000000000000000 ) ) ;
#59518=CARTESIAN_POINT ( 'NONE',  ( 165.2494399300530290, -11.64849832608277325, -3.999999999999998224 ) ) ;
#59519=CARTESIAN_POINT ( 'NONE',  ( -23.40286736638519471, -122.5496321078137356, 22.50000000000000000 ) ) ;
#59524=FACE_OUTER_BOUND ( 'NONE', #58433, .T. ) ;
#59551=FACE_BOUND ( 'NONE', #86222, .T. ) ;
#59552=CIRCLE ( 'NONE', #42906, 11.68950434577434372 ) ;
#59626=CIRCLE ( 'NONE', #55076, 204.9779373800640485 ) ;
#59633=CIRCLE ( 'NONE', #68673, 1.000000000000000888 ) ;
#59652=CIRCLE ( 'NONE', #18808, 7.999999999999998224 ) ;
#59658=AXIS2_PLACEMENT_3D ( 'NONE', #46928, #46012, #75372 ) ;
#59688=EDGE_CURVE ( 'NONE', #74706, #46033, #54957, .T. ) ;
#59704=CIRCLE ( 'NONE', #39990, 1.000000000000000888 ) ;
#59750=CARTESIAN_POINT ( 'NONE',  ( -36.09237171215955442, -122.5496321078137356, -21.50000000000000000 ) ) ;
#59774=CARTESIAN_POINT ( 'NONE',  ( 73.43068321062709458, -134.2391364535880598, 0.000000000000000000 ) ) ;
#59793=DIRECTION ( 'NONE',  ( -0.000000000000000000, 1.000000000000000000, -0.000000000000000000 ) ) ;
#59820=ORIENTED_EDGE ( 'NONE', *, *, #48813, .F. ) ;
#59842=VERTEX_POINT ( 'NONE', #61157 ) ;
#59856=AXIS2_PLACEMENT_3D ( 'NONE', #66573, #74125, #7404 ) ;
#59890=DIRECTION ( 'NONE',  ( -0.000000000000000000, 1.000000000000000000, -0.000000000000000000 ) ) ;
#59950=ADVANCED_FACE ( 'NONE', ( #75339 ), #82889, .T. ) ;
#59954=FACE_OUTER_BOUND ( 'NONE', #68254, .T. ) ;
#59960=ORIENTED_EDGE ( 'NONE', *, *, #1142, .T. ) ;
#59975=CARTESIAN_POINT ( 'NONE',  ( 123.4306832106270946, -134.2641364535880939, 4.999999999999990230 ) ) ;
#60076=EDGE_LOOP ( 'NONE', ( #78289, #91587, #25569 ) ) ;
#60125=ADVANCED_FACE ( 'NONE', ( #16538 ), #45392, .T. ) ;
#60194=FACE_OUTER_BOUND ( 'NONE', #82034, .T. ) ;
#60207=FACE_OUTER_BOUND ( 'NONE', #35504, .T. ) ;
#60229=EDGE_CURVE ( 'NONE', #93421, #40890, #10819, .T. ) ;
#60290=VERTEX_POINT ( 'NONE', #54840 ) ;
#60302=ORIENTED_EDGE ( 'NONE', *, *, #30492, .T. ) ;
#60305=AXIS2_PLACEMENT_3D ( 'NONE', #40023, #62793, #40475 ) ;
#60315=CARTESIAN_POINT ( 'NONE',  ( 194.7510731661265595, -164.3527196417747405, -21.50000000000000000 ) ) ;
#60326=DIRECTION ( 'NONE',  ( -1.000000000000000000, 0.000000000000000000, 0.000000000000000000 ) ) ;
#60350=FACE_OUTER_BOUND ( 'NONE', #87608, .T. ) ;
#60407=VERTEX_POINT ( 'NONE', #63397 ) ;
#60436=CARTESIAN_POINT ( 'NONE',  ( 222.4306832106270804, -141.7221692137691775, -21.50000000000000000 ) ) ;
#60446=FACE_OUTER_BOUND ( 'NONE', #48586, .T. ) ;
#60464=CYLINDRICAL_SURFACE ( 'NONE', #54791, 1.000000000000000888 ) ;
#60489=VERTEX_POINT ( 'NONE', #4661 ) ;
#60503=VECTOR ( 'NONE', #7522, 1000.000000000000000 ) ;
#60534=EDGE_LOOP ( 'NONE', ( #47220, #69587, #21164, #8202 ) ) ;
#60561=CYLINDRICAL_SURFACE ( 'NONE', #33646, 204.9779373800640485 ) ;
#60629=ORIENTED_EDGE ( 'NONE', *, *, #92477, .F. ) ;
#60651=ADVANCED_FACE ( 'NONE', ( #41565, #70488 ), #85600, .F. ) ;
#60666=EDGE_CURVE ( 'NONE', #70970, #43675, #13999, .T. ) ;
#60693=CARTESIAN_POINT ( 'NONE',  ( 123.4306832106270946, -178.2391364535880882, 0.000000000000000000 ) ) ;
#60743=LINE ( 'NONE', #39392, #41480 ) ;
#60760=ORIENTED_EDGE ( 'NONE', *, *, #40423, .F. ) ;
#60761=ADVANCED_FACE ( 'NONE', ( #51011 ), #79898, .T. ) ;
#60794=CARTESIAN_POINT ( 'NONE',  ( -23.40286736638519471, -122.5496321078137356, 21.50000000000000000 ) ) ;
#60845=VERTEX_POINT ( 'NONE', #7014 ) ;
#60988=DIRECTION ( 'NONE',  ( 0.000000000000000000, 0.000000000000000000, -1.000000000000000000 ) ) ;
#60992=CARTESIAN_POINT ( 'NONE',  ( 194.5881128153457098, 0.000000000000000000, 10.00000000000000178 ) ) ;
#61007=DIRECTION ( 'NONE',  ( 0.000000000000000000, 0.000000000000000000, 1.000000000000000000 ) ) ;
#61078=DIRECTION ( 'NONE',  ( 0.000000000000000000, 0.000000000000000000, 1.000000000000000000 ) ) ;
#61083=EDGE_CURVE ( 'NONE', #14651, #74347, #12434, .T. ) ;
#61089=ADVANCED_FACE ( 'NONE', ( #89299 ), #62389, .T. ) ;
#61106=ORIENTED_EDGE ( 'NONE', *, *, #78869, .T. ) ;
#61107=AXIS2_PLACEMENT_3D ( 'NONE', #30970, #43755, #8249 ) ;
#61113=CARTESIAN_POINT ( 'NONE',  ( 60.83289261295100658, -250.0118895884541530, 22.50000000000000000 ) ) ;
#61119=VECTOR ( 'NONE', #70114, 1000.000000000000000 ) ;
#61125=ORIENTED_EDGE ( 'NONE', *, *, #61083, .F. ) ;
#61126=DIRECTION ( 'NONE',  ( 0.000000000000000000, 0.7071067811867438602, 0.7071067811863512853 ) ) ;
#61128=TOROIDAL_SURFACE ( 'NONE', #67128, 16.36528803885689243, 1.000000000000000000 ) ;
#61157=CARTESIAN_POINT ( 'NONE',  ( 73.43068321062709458, -134.2391364535880598, -5.025000000000002132 ) ) ;
#61165=ADVANCED_FACE ( 'NONE', ( #81742 ), #27582, .T. ) ;
#61188=ADVANCED_FACE ( 'NONE', ( #52864 ), #16892, .T. ) ;
#61204=CONICAL_SURFACE ( 'NONE', #14374, 4.000000000000003553, 1.029744258676654534 ) ;
#61209=VERTEX_POINT ( 'NONE', #31115 ) ;
#61220=VERTEX_POINT ( 'NONE', #68960 ) ;
#61232=EDGE_LOOP ( 'NONE', ( #31379, #49116, #4562, #1694 ) ) ;
#61255=CARTESIAN_POINT ( 'NONE',  ( -23.40286736638519471, -134.2391364535880598, -21.50000000000000000 ) ) ;
#61271=DIRECTION ( 'NONE',  ( 0.000000000000000000, 0.000000000000000000, 1.000000000000000000 ) ) ;
#61293=CARTESIAN_POINT ( 'NONE',  ( 139.6925840978351232, -135.2391364535880882, 22.50000000000000000 ) ) ;
#61339=ADVANCED_FACE ( 'NONE', ( #2693 ), #60464, .T. ) ;
#61477=ORIENTED_EDGE ( 'NONE', *, *, #73959, .F. ) ;
#61500=FACE_OUTER_BOUND ( 'NONE', #91414, .T. ) ;
#61524=ORIENTED_EDGE ( 'NONE', *, *, #83427, .T. ) ;
#61569=DIRECTION ( 'NONE',  ( -1.000000000000000000, 0.000000000000000000, 0.000000000000000000 ) ) ;
#61589=DIRECTION ( 'NONE',  ( -0.000000000000000000, -0.000000000000000000, 1.000000000000000000 ) ) ;
#61613=FACE_OUTER_BOUND ( 'NONE', #44411, .T. ) ;
#61626=ORIENTED_EDGE ( 'NONE', *, *, #56487, .T. ) ;
#61642=FACE_OUTER_BOUND ( 'NONE', #4941, .T. ) ;
#61663=( LENGTH_UNIT ( ) NAMED_UNIT ( * ) SI_UNIT ( .MILLI., .METRE. ) );
#61710=CYLINDRICAL_SURFACE ( 'NONE', #70238, 7.999999999999992895 ) ;
#61742=ORIENTED_EDGE ( 'NONE', *, *, #33379, .T. ) ;
#61868=ORIENTED_EDGE ( 'NONE', *, *, #39228, .F. ) ;
#61883=FACE_OUTER_BOUND ( 'NONE', #88462, .T. ) ;
#61953=ADVANCED_FACE ( 'NONE', ( #87505 ), #22652, .T. ) ;
#61955=EDGE_CURVE ( 'NONE', #83166, #37793, #81804, .T. ) ;
#61989=ORIENTED_EDGE ( 'NONE', *, *, #87285, .T. ) ;
#62017=EDGE_CURVE ( 'NONE', #10408, #3537, #38224, .T. ) ;
#62037=ORIENTED_EDGE ( 'NONE', *, *, #51756, .T. ) ;
#62074=DIRECTION ( 'NONE',  ( 1.000000000000000000, 0.000000000000000000, 0.000000000000000000 ) ) ;
#62075=CARTESIAN_POINT ( 'NONE',  ( 123.4306832106270946, -134.2391364535880882, 5.024999999999987921 ) ) ;
#62105=PLANE ( 'NONE',  #23920 ) ;
#62171=DIRECTION ( 'NONE',  ( -1.000000000000000000, 1.124465274301078034E-16, 0.000000000000000000 ) ) ;
#62192=PLANE ( 'NONE',  #84529 ) ;
#62211=DIRECTION ( 'NONE',  ( 0.000000000000000000, 1.000000000000000000, 0.000000000000000000 ) ) ;
#62226=DIRECTION ( 'NONE',  ( 0.000000000000000000, 0.000000000000000000, 1.000000000000000000 ) ) ;
#62263=VECTOR ( 'NONE', #828, 1000.000000000000000 ) ;
#62313=CIRCLE ( 'NONE', #24445, 1.000000000000000888 ) ;
#62357=ADVANCED_FACE ( 'NONE', ( #6959 ), #78462, .F. ) ;
#62389=TOROIDAL_SURFACE ( 'NONE', #86555, 160.1282194813176716, 1.000000000000000000 ) ;
#62396=( GEOMETRIC_REPRESENTATION_CONTEXT ( 3 ) GLOBAL_UNCERTAINTY_ASSIGNED_CONTEXT ( ( #25414 ) ) GLOBAL_UNIT_ASSIGNED_CONTEXT ( ( #24432, #51915, #52845 ) ) REPRESENTATION_CONTEXT ( 'NONE', 'WORKASPACE' ) );
#62447=CIRCLE ( 'NONE', #9555, 7.500000000000012434 ) ;
#62453=CARTESIAN_POINT ( 'NONE',  ( 17.06571399127465583, -89.54582641780471874, 21.50000000000000000 ) ) ;
#62463=AXIS2_PLACEMENT_3D ( 'NONE', #59519, #8822, #45261 ) ;
#62520=DIRECTION ( 'NONE',  ( 0.000000000000000000, 0.000000000000000000, 1.000000000000000000 ) ) ;
#62551=AXIS2_PLACEMENT_3D ( 'NONE', #74658, #9782, #39104 ) ;
#62559=TOROIDAL_SURFACE ( 'NONE', #71697, 154.4364916446740210, 1.000000000000000000 ) ;
#62588=DIRECTION ( 'NONE',  ( 1.000000000000000000, 0.000000000000000000, 0.000000000000000000 ) ) ;
#62606=ORIENTED_EDGE ( 'NONE', *, *, #31797, .F. ) ;
#62615=SHAPE_REPRESENTATION_RELATIONSHIP ( 'NONE' , 'NONE' ,  #42162, #88142 ) ;
#62623=AXIS2_PLACEMENT_3D ( 'NONE', #19422, #27465, #19886 ) ;
#62628=DIRECTION ( 'NONE',  ( 0.000000000000000000, 0.000000000000000000, 1.000000000000000000 ) ) ;
#62679=CIRCLE ( 'NONE', #70244, 0.9999999999999977796 ) ;
#62704=ORIENTED_EDGE ( 'NONE', *, *, #40665, .T. ) ;
#62764=ORIENTED_EDGE ( 'NONE', *, *, #2175, .F. ) ;
#62766=UNCERTAINTY_MEASURE_WITH_UNIT (LENGTH_MEASURE( 1.000000000000000082E-05 ), #61663, 'distance_accuracy_value', 'NONE');
#62793=DIRECTION ( 'NONE',  ( 1.000000000000000000, 0.000000000000000000, 0.000000000000000000 ) ) ;
#62815=DIRECTION ( 'NONE',  ( 1.000000000000000000, 0.000000000000000000, 0.000000000000000000 ) ) ;
#62873=DIRECTION ( 'NONE',  ( 1.000000000000000000, -0.000000000000000000, -0.000000000000000000 ) ) ;
#62885=ORIENTED_EDGE ( 'NONE', *, *, #19944, .F. ) ;
#62925=ADVANCED_FACE ( 'NONE', ( #18125 ), #82092, .T. ) ;
#62957=ORIENTED_EDGE ( 'NONE', *, *, #90893, .F. ) ;
#62965=DIRECTION ( 'NONE',  ( -1.000000000000000000, 1.124465274301078034E-16, 0.000000000000000000 ) ) ;
#62997=EDGE_CURVE ( 'NONE', #58890, #6488, #76021, .T. ) ;
#63066=CARTESIAN_POINT ( 'NONE',  ( -147.8070425842520308, 32.24468615100210656, 21.50000000000000000 ) ) ;
#63100=DIRECTION ( 'NONE',  ( -0.000000000000000000, -0.000000000000000000, -1.000000000000000000 ) ) ;
#63113=ORIENTED_EDGE ( 'NONE', *, *, #44097, .F. ) ;
#63125=DIRECTION ( 'NONE',  ( -1.000000000000000000, 0.000000000000000000, 0.000000000000000000 ) ) ;
#63131=DIRECTION ( 'NONE',  ( 0.000000000000000000, 0.000000000000000000, 1.000000000000000000 ) ) ;
#63264=DIRECTION ( 'NONE',  ( 0.000000000000000000, 0.000000000000000000, 1.000000000000000000 ) ) ;
#63339=EDGE_LOOP ( 'NONE', ( #3448, #56200, #40420, #39053 ) ) ;
#63349=EDGE_CURVE ( 'NONE', #66913, #4348, #79086, .T. ) ;
#63350=DIRECTION ( 'NONE',  ( -1.000000000000000000, 0.000000000000000000, 0.000000000000000000 ) ) ;
#63355=VERTEX_POINT ( 'NONE', #11950 ) ;
#63387=DIRECTION ( 'NONE',  ( -0.000000000000000000, -0.000000000000000000, -1.000000000000000000 ) ) ;
#63397=CARTESIAN_POINT ( 'NONE',  ( -186.9122233887894140, -89.54582641780471874, -22.50000000000000000 ) ) ;
#63462=EDGE_CURVE ( 'NONE', #67590, #67510, #69252, .T. ) ;
#63480=DIRECTION ( 'NONE',  ( 1.000000000000000000, 0.000000000000000000, 0.000000000000000000 ) ) ;
#63494=SPHERICAL_SURFACE ( 'NONE', #55082, 1.000000000000000000 ) ;
#63505=EDGE_CURVE ( 'NONE', #75656, #90187, #68178, .T. ) ;
#63524=FACE_OUTER_BOUND ( 'NONE', #64615, .T. ) ;
#63710=CARTESIAN_POINT ( 'NONE',  ( -147.0026986695707762, -210.7421749798627388, 22.50000000000000000 ) ) ;
#63730=DIRECTION ( 'NONE',  ( -0.000000000000000000, -1.000000000000000000, -0.000000000000000000 ) ) ;
#63778=VERTEX_POINT ( 'NONE', #27096 ) ;
#63788=DIRECTION ( 'NONE',  ( -1.000000000000000000, 0.000000000000000000, 0.000000000000000000 ) ) ;
#63808=DIRECTION ( 'NONE',  ( 1.000000000000000000, 0.000000000000000000, 0.000000000000000000 ) ) ;
#63815=DIRECTION ( 'NONE',  ( -0.000000000000000000, -0.000000000000000000, 1.000000000000000000 ) ) ;
#63830=VECTOR ( 'NONE', #86466, 1000.000000000000000 ) ;
#63899=AXIS2_PLACEMENT_3D ( 'NONE', #87299, #35740, #93020 ) ;
#63937=ORIENTED_EDGE ( 'NONE', *, *, #50938, .T. ) ;
#63976=AXIS2_PLACEMENT_3D ( 'NONE', #83677, #55755, #55292 ) ;
#64053=AXIS2_PLACEMENT_3D ( 'NONE', #53072, #66827, #89985 ) ;
#64107=AXIS2_PLACEMENT_3D ( 'NONE', #3220, #19763, #61007 ) ;
#64112=ORIENTED_EDGE ( 'NONE', *, *, #70761, .F. ) ;
#64190=CIRCLE ( 'NONE', #83792, 161.1282194813176716 ) ;
#64195=AXIS2_PLACEMENT_3D ( 'NONE', #41070, #63387, #48664 ) ;
#64203=AXIS2_PLACEMENT_3D ( 'NONE', #41282, #13385, #63125 ) ;
#64210=CIRCLE ( 'NONE', #47518, 1.000000000000002887 ) ;
#64250=EDGE_CURVE ( 'NONE', #27807, #18158, #9966, .T. ) ;
#64291=VECTOR ( 'NONE', #25535, 1000.000000000000114 ) ;
#64336=ADVANCED_FACE ( 'NONE', ( #2871 ), #23719, .T. ) ;
#64437=CARTESIAN_POINT ( 'NONE',  ( 222.4306832106270804, -135.2391364535880882, -21.50000000000000000 ) ) ;
#64449=DIRECTION ( 'NONE',  ( -1.000000000000000000, 2.640448681563344014E-15, 0.000000000000000000 ) ) ;
#64549=ADVANCED_FACE ( 'NONE', ( #31755 ), #89485, .T. ) ;
#64552=ORIENTED_EDGE ( 'NONE', *, *, #1420, .T. ) ;
#64615=EDGE_LOOP ( 'NONE', ( #27088, #44714, #26265, #75169 ) ) ;
#64618=EDGE_LOOP ( 'NONE', ( #60760, #70039 ) ) ;
#64761=CARTESIAN_POINT ( 'NONE',  ( 180.7149167944524493, -12.49482340714361506, -3.999999999999998224 ) ) ;
#64800=DIRECTION ( 'NONE',  ( -0.8429829950866658539, -0.5379402104274361163, 3.232101055797385739E-15 ) ) ;
#64807=DIRECTION ( 'NONE',  ( -0.000000000000000000, -0.000000000000000000, -1.000000000000000000 ) ) ;
#64907=DIRECTION ( 'NONE',  ( -0.000000000000000000, -1.000000000000000000, -0.000000000000000000 ) ) ;
#64968=ORIENTED_EDGE ( 'NONE', *, *, #56487, .F. ) ;
#65037=LINE ( 'NONE', #21447, #4964 ) ;
#65039=ORIENTED_EDGE ( 'NONE', *, *, #80951, .T. ) ;
#65047=ORIENTED_EDGE ( 'NONE', *, *, #45328, .F. ) ;
#65131=ADVANCED_FACE ( 'NONE', ( #19413 ), #42839, .F. ) ;
#65204=EDGE_LOOP ( 'NONE', ( #65909, #19637, #61125 ) ) ;
#65232=CARTESIAN_POINT ( 'NONE',  ( 139.6925840978351516, 15.36528803885690664, 22.50000000000000000 ) ) ;
#65251=VECTOR ( 'NONE', #31144, 1000.000000000000000 ) ;
#65254=DIRECTION ( 'NONE',  ( -0.5379402104274313423, 0.8429829950866690735, 0.000000000000000000 ) ) ;
#65272=CARTESIAN_POINT ( 'NONE',  ( -22.78264641048746597, -118.9815703160634541, -21.50000000000000000 ) ) ;
#65298=CARTESIAN_POINT ( 'NONE',  ( -23.68628624284178130, -43.55766379199612004, 21.50000000000000000 ) ) ;
#65302=EDGE_LOOP ( 'NONE', ( #46725, #69362, #11057, #26408 ) ) ;
#65310=EDGE_LOOP ( 'NONE', ( #77485, #62885, #47889, #81880 ) ) ;
#65458=AXIS2_PLACEMENT_3D ( 'NONE', #37252, #45260, #73711 ) ;
#65478=AXIS2_PLACEMENT_3D ( 'NONE', #26571, #55459, #47859 ) ;
#65497=VERTEX_POINT ( 'NONE', #79974 ) ;
#65504=ORIENTED_EDGE ( 'NONE', *, *, #67502, .T. ) ;
#65507=CIRCLE ( 'NONE', #18635, 0.9999999999999985567 ) ;
#65521=CIRCLE ( 'NONE', #24661, 7.500000000000012434 ) ;
#65538=EDGE_CURVE ( 'NONE', #41863, #29328, #5067, .T. ) ;
#65548=CIRCLE ( 'NONE', #14167, 7.999999999999992895 ) ;
#65566=ORIENTED_EDGE ( 'NONE', *, *, #33379, .F. ) ;
#65654=VECTOR ( 'NONE', #18844, 1000.000000000000000 ) ;
#65681=VECTOR ( 'NONE', #19941, 1000.000000000000000 ) ;
#65682=DIRECTION ( 'NONE',  ( 1.000000000000000000, 0.000000000000000000, 0.000000000000000000 ) ) ;
#65699=LINE ( 'NONE', #89625, #45813 ) ;
#65716=CARTESIAN_POINT ( 'NONE',  ( 222.8344101925596306, 0.000000000000000000, 21.50000000000000000 ) ) ;
#65740=CONICAL_SURFACE ( 'NONE', #86850, 4.000000000000003553, 1.029744258676654534 ) ;
#65744=ORIENTED_EDGE ( 'NONE', *, *, #88395, .T. ) ;
#65757=ORIENTED_EDGE ( 'NONE', *, *, #87153, .F. ) ;
#65824=VECTOR ( 'NONE', #42448, 1000.000000000000000 ) ;
#65831=CARTESIAN_POINT ( 'NONE',  ( 194.7510731661265595, -143.7221692137691775, 22.50000000000000000 ) ) ;
#65874=DIRECTION ( 'NONE',  ( 1.000000000000000000, 0.000000000000000000, 0.000000000000000000 ) ) ;
#65909=ORIENTED_EDGE ( 'NONE', *, *, #22374, .T. ) ;
#65910=ADVANCED_FACE ( 'NONE', ( #16967 ), #37794, .F. ) ;
#65942=DIRECTION ( 'NONE',  ( 0.000000000000000000, 1.000000000000000000, 0.000000000000000000 ) ) ;
#65961=CARTESIAN_POINT ( 'NONE',  ( 196.7510731661265595, -143.7221692137691775, -32.50000000000000711 ) ) ;
#65973=CARTESIAN_POINT ( 'NONE',  ( 2.197429475817664013, -229.5268262511776527, 22.50000000000000000 ) ) ;
#65993=EDGE_LOOP ( 'NONE', ( #15740, #53740, #5309, #76183 ) ) ;
#66045=DIRECTION ( 'NONE',  ( -1.000000000000000000, 0.000000000000000000, 0.000000000000000000 ) ) ;
#66092=CIRCLE ( 'NONE', #28235, 7.999999999999998224 ) ;
#66129=CARTESIAN_POINT ( 'NONE',  ( 61.37083282337847123, -250.8548725835408391, 21.50000000000000000 ) ) ;
#66174=CARTESIAN_POINT ( 'NONE',  ( 194.7510731661265595, -142.7221692137691775, -21.50000000000000000 ) ) ;
#66210=CARTESIAN_POINT ( 'NONE',  ( 143.6449502718966755, -26.00396092263537540, -47.19625681453479871 ) ) ;
#66220=EDGE_CURVE ( 'NONE', #57488, #44867, #25922, .T. ) ;
#66246=ORIENTED_EDGE ( 'NONE', *, *, #2847, .F. ) ;
#66262=CARTESIAN_POINT ( 'NONE',  ( 123.4306832106270946, -134.2391364535880882, -4.999999999999990230 ) ) ;
#66299=ORIENTED_EDGE ( 'NONE', *, *, #66834, .F. ) ;
#66306=ADVANCED_FACE ( 'NONE', ( #5105 ), #26874, .F. ) ;
#66365=DIRECTION ( 'NONE',  ( 1.000000000000000000, 0.000000000000000000, 0.000000000000000000 ) ) ;
#66378=LINE ( 'NONE', #30379, #29273 ) ;
#66386=CARTESIAN_POINT ( 'NONE',  ( 222.4306832106270804, -142.7221692137691775, -21.50000000000000000 ) ) ;
#66498=FACE_OUTER_BOUND ( 'NONE', #87863, .T. ) ;
#66517=VECTOR ( 'NONE', #72213, 1000.000000000000000 ) ;
#66549=ORIENTED_EDGE ( 'NONE', *, *, #92592, .T. ) ;
#66573=CARTESIAN_POINT ( 'NONE',  ( -23.68628624284178130, -55.96374926131388605, -22.50000000000000000 ) ) ;
#66594=PLANE ( 'NONE',  #71523 ) ;
#66676=ADVANCED_FACE ( 'NONE', ( #28745 ), #73131, .T. ) ;
#66700=ORIENTED_EDGE ( 'NONE', *, *, #8700, .T. ) ;
#66715=CARTESIAN_POINT ( 'NONE',  ( 208.4306832106271088, -44.55766379199612004, -7.500000000000012434 ) ) ;
#66730=DIRECTION ( 'NONE',  ( 0.000000000000000000, 0.7071067811865474617, 0.7071067811865474617 ) ) ;
#66772=AXIS2_PLACEMENT_3D ( 'NONE', #66955, #87315, #88712 ) ;
#66827=DIRECTION ( 'NONE',  ( 1.124465274301078281E-16, 1.000000000000000000, -0.000000000000000000 ) ) ;
#66834=EDGE_CURVE ( 'NONE', #50388, #6488, #6037, .T. ) ;
#66857=CARTESIAN_POINT ( 'NONE',  ( 222.4306832106270804, -134.2391364535880882, -21.50000000000000000 ) ) ;
#66913=VERTEX_POINT ( 'NONE', #64761 ) ;
#66936=CARTESIAN_POINT ( 'NONE',  ( 195.7510731661265595, -164.3527196417747405, 21.50000000000000000 ) ) ;
#66955=CARTESIAN_POINT ( 'NONE',  ( 196.7510731661265595, -143.7221692137691775, 21.50000000000000000 ) ) ;
#66975=LINE ( 'NONE', #61293, #72664 ) ;
#66977=AXIS2_PLACEMENT_3D ( 'NONE', #52008, #82291, #22660 ) ;
#67000=AXIS2_PLACEMENT_3D ( 'NONE', #17817, #10696, #75574 ) ;
#67029=ORIENTED_EDGE ( 'NONE', *, *, #16816, .T. ) ;
#67043=DIRECTION ( 'NONE',  ( -1.000000000000000000, 0.000000000000000000, 0.000000000000000000 ) ) ;
#67098=CARTESIAN_POINT ( 'NONE',  ( -18.20453976106250948, -63.49190233628851132, 21.50000000000000000 ) ) ;
#67125=ORIENTED_EDGE ( 'NONE', *, *, #69736, .F. ) ;
#67128=AXIS2_PLACEMENT_3D ( 'NONE', #69522, #90794, #25953 ) ;
#67180=EDGE_CURVE ( 'NONE', #75708, #92063, #86759, .T. ) ;
#67207=DIRECTION ( 'NONE',  ( -1.000000000000000000, 8.612884727757786904E-16, 0.000000000000000000 ) ) ;
#67209=LINE ( 'NONE', #1391, #21789 ) ;
#67222=DIRECTION ( 'NONE',  ( -1.000000000000000000, 0.000000000000000000, 0.000000000000000000 ) ) ;
#67234=DIRECTION ( 'NONE',  ( -0.000000000000000000, -0.000000000000000000, -1.000000000000000000 ) ) ;
#67285=AXIS2_PLACEMENT_3D ( 'NONE', #50022, #86457, #13142 ) ;
#67335=ORIENTED_EDGE ( 'NONE', *, *, #87153, .T. ) ;
#67454=CARTESIAN_POINT ( 'NONE',  ( -23.68628624284178130, -44.55766379199612004, 22.50000000000000000 ) ) ;
#67502=EDGE_CURVE ( 'NONE', #82047, #12908, #59552, .T. ) ;
#67510=VERTEX_POINT ( 'NONE', #67522 ) ;
#67522=CARTESIAN_POINT ( 'NONE',  ( 222.4306832106270804, -141.7221692137691775, 22.50000000000000000 ) ) ;
#67590=VERTEX_POINT ( 'NONE', #33383 ) ;
#67591=DIRECTION ( 'NONE',  ( -1.000000000000000000, 0.000000000000000000, 0.000000000000000000 ) ) ;
#67607=ORIENTED_EDGE ( 'NONE', *, *, #51429, .T. ) ;
#67620=DIRECTION ( 'NONE',  ( -0.000000000000000000, -0.000000000000000000, 1.000000000000000000 ) ) ;
#67622=EDGE_CURVE ( 'NONE', #85761, #4348, #26287, .T. ) ;
#67624=CARTESIAN_POINT ( 'NONE',  ( 200.9306832106271088, -142.7221692137691775, 0.000000000000000000 ) ) ;
#67708=DIRECTION ( 'NONE',  ( 0.000000000000000000, 0.000000000000000000, 1.000000000000000000 ) ) ;
#67726=EDGE_LOOP ( 'NONE', ( #85779, #75871, #66299, #89831 ) ) ;
#67779=CARTESIAN_POINT ( 'NONE',  ( -36.09237171215956863, 15.36528803885690664, 22.50000000000000000 ) ) ;
#67789=CIRCLE ( 'NONE', #60305, 1.000000000000000888 ) ;
#67856=EDGE_LOOP ( 'NONE', ( #53021, #86648, #87220, #66549 ) ) ;
#67992=CARTESIAN_POINT ( 'NONE',  ( -39.80257052418233599, -229.5268262511776527, 22.47499999999998721 ) ) ;
#68037=DIRECTION ( 'NONE',  ( -0.8457827187922973833, -0.5335274993777826547, 0.000000000000000000 ) ) ;
#68138=CARTESIAN_POINT ( 'NONE',  ( 221.8344101925596306, -43.55766379199612004, 22.50000000000000000 ) ) ;
#68170=CARTESIAN_POINT ( 'NONE',  ( 73.43068321062709458, -134.2391364535880598, 0.000000000000000000 ) ) ;
#68178=( BOUNDED_CURVE ( )  B_SPLINE_CURVE ( 3, ( #4380, #70667, #5796, #41271 ),
 .UNSPECIFIED., .F., .T. ) 
 B_SPLINE_CURVE_WITH_KNOTS ( ( 4, 4 ),
 ( 3.141592653589793116, 4.712388980384689674 ),
 .UNSPECIFIED. ) 
 CURVE ( )  GEOMETRIC_REPRESENTATION_ITEM ( )  RATIONAL_B_SPLINE_CURVE ( ( 1.000000000000000000, 0.8047378541243649375, 0.8047378541243649375, 1.000000000000000000 ) ) 
 REPRESENTATION_ITEM ( '' )  );
#68241=DIRECTION ( 'NONE',  ( 0.000000000000000000, 0.000000000000000000, 1.000000000000000000 ) ) ;
#68254=EDGE_LOOP ( 'NONE', ( #6856, #45084, #69244, #47670 ) ) ;
#68259=DIRECTION ( 'NONE',  ( 0.000000000000000000, 0.000000000000000000, -1.000000000000000000 ) ) ;
#68271=DIRECTION ( 'NONE',  ( 0.000000000000000000, 1.000000000000000000, 0.000000000000000000 ) ) ;
#68273=DIRECTION ( 'NONE',  ( -0.000000000000000000, -0.000000000000000000, 1.000000000000000000 ) ) ;
#68351=CARTESIAN_POINT ( 'NONE',  ( 123.4306832106270946, -134.2391364535880882, 0.000000000000000000 ) ) ;
#68411=ORIENTED_EDGE ( 'NONE', *, *, #24610, .T. ) ;
#68437=CYLINDRICAL_SURFACE ( 'NONE', #75952, 4.000000000000003553 ) ;
#68456=AXIS2_PLACEMENT_3D ( 'NONE', #47207, #39628, #54790 ) ;
#68501=ORIENTED_EDGE ( 'NONE', *, *, #27196, .T. ) ;
#68553=CIRCLE ( 'NONE', #67000, 1.000000000000000888 ) ;
#68560=EDGE_CURVE ( 'NONE', #3498, #15284, #88311, .T. ) ;
#68581=DIRECTION ( 'NONE',  ( -1.000000000000000000, 0.000000000000000000, 0.000000000000000000 ) ) ;
#68596=DIRECTION ( 'NONE',  ( -0.000000000000000000, -0.000000000000000000, -1.000000000000000000 ) ) ;
#68602=DIRECTION ( 'NONE',  ( -0.000000000000000000, -0.000000000000000000, -1.000000000000000000 ) ) ;
#68619=AXIS2_PLACEMENT_3D ( 'NONE', #41189, #32726, #68241 ) ;
#68642=DIRECTION ( 'NONE',  ( 0.000000000000000000, 0.000000000000000000, 1.000000000000000000 ) ) ;
#68673=AXIS2_PLACEMENT_3D ( 'NONE', #89403, #2340, #37821 ) ;
#68679=VERTEX_POINT ( 'NONE', #7776 ) ;
#68682=VECTOR ( 'NONE', #66730, 1000.000000000000114 ) ;
#68690=CYLINDRICAL_SURFACE ( 'NONE', #27883, 1.000000000000000888 ) ;
#68758=AXIS2_PLACEMENT_3D ( 'NONE', #85075, #35368, #63808 ) ;
#68768=EDGE_CURVE ( 'NONE', #79604, #72125, #80753, .T. ) ;
#68769=DIRECTION ( 'NONE',  ( -0.000000000000000000, 1.000000000000000000, -0.000000000000000000 ) ) ;
#68781=DIRECTION ( 'NONE',  ( 0.000000000000000000, 0.000000000000000000, 1.000000000000000000 ) ) ;
#68798=ORIENTED_EDGE ( 'NONE', *, *, #41200, .F. ) ;
#68866=DIRECTION ( 'NONE',  ( 0.000000000000000000, 0.000000000000000000, -1.000000000000000000 ) ) ;
#68908=EDGE_CURVE ( 'NONE', #5915, #93421, #59626, .T. ) ;
#68920=CARTESIAN_POINT ( 'NONE',  ( 188.7149167944524493, -12.49482340714361506, -3.999999999999998224 ) ) ;
#68957=CARTESIAN_POINT ( 'NONE',  ( 223.4306832106270804, -134.2391364535880882, -21.50000000000000000 ) ) ;
#68960=CARTESIAN_POINT ( 'NONE',  ( -36.09237171215954021, -122.5496321078137356, 22.50000000000000000 ) ) ;
#68962=AXIS2_PLACEMENT_3D ( 'NONE', #65298, #80390, #87029 ) ;
#68972=EDGE_CURVE ( 'NONE', #26019, #90518, #38426, .T. ) ;
#69050=DIRECTION ( 'NONE',  ( 0.000000000000000000, 1.000000000000000000, 0.000000000000000000 ) ) ;
#69069=EDGE_CURVE ( 'NONE', #4348, #66913, #33922, .T. ) ;
#69100=CARTESIAN_POINT ( 'NONE',  ( -23.68628624284178130, -55.96374926131388605, 21.50000000000000000 ) ) ;
#69157=ADVANCED_FACE ( 'NONE', ( #3002 ), #61710, .F. ) ;
#69238=DIRECTION ( 'NONE',  ( 0.000000000000000000, 0.000000000000000000, 1.000000000000000000 ) ) ;
#69244=ORIENTED_EDGE ( 'NONE', *, *, #82386, .T. ) ;
#69252=LINE ( 'NONE', #84837, #45790 ) ;
#69303=CARTESIAN_POINT ( 'NONE',  ( 123.4306832106270946, -178.2391364535880882, 0.000000000000000000 ) ) ;
#69360=ORIENTED_EDGE ( 'NONE', *, *, #87626, .T. ) ;
#69362=ORIENTED_EDGE ( 'NONE', *, *, #7047, .F. ) ;
#69405=CIRCLE ( 'NONE', #8902, 11.68950434577434372 ) ;
#69432=ORIENTED_EDGE ( 'NONE', *, *, #27196, .F. ) ;
#69474=CARTESIAN_POINT ( 'NONE',  ( 215.9306832106270804, -324.2391364535881735, 9.184850993605165694E-16 ) ) ;
#69477=CONICAL_SURFACE ( 'NONE', #28665, 5.024999999999987921, 0.7853981633974482790 ) ;
#69481=CONICAL_SURFACE ( 'NONE', #40715, 4.000000000000003553, 1.029744258676654534 ) ;
#69522=CARTESIAN_POINT ( 'NONE',  ( 139.6925840978351516, 15.36528803885690664, -21.50000000000000000 ) ) ;
#69544=VECTOR ( 'NONE', #20023, 1000.000000000000114 ) ;
#69555=ORIENTED_EDGE ( 'NONE', *, *, #43643, .T. ) ;
#69587=ORIENTED_EDGE ( 'NONE', *, *, #89784, .F. ) ;
#69603=ORIENTED_EDGE ( 'NONE', *, *, #73898, .F. ) ;
#69642=DIRECTION ( 'NONE',  ( -0.000000000000000000, -0.000000000000000000, -1.000000000000000000 ) ) ;
#69656=DIRECTION ( 'NONE',  ( 0.8043439146810466012, 0.5941640067486159138, 0.000000000000000000 ) ) ;
#69727=CARTESIAN_POINT ( 'NONE',  ( -23.40286736638519471, -135.2391364535880598, -21.50000000000000000 ) ) ;
#69736=EDGE_CURVE ( 'NONE', #34073, #23241, #62447, .T. ) ;
#69816=AXIS2_PLACEMENT_3D ( 'NONE', #1245, #75890, #30127 ) ;
#69826=ORIENTED_EDGE ( 'NONE', *, *, #9644, .T. ) ;
#69834=EDGE_CURVE ( 'NONE', #41591, #12908, #50656, .T. ) ;
#69889=AXIS2_PLACEMENT_3D ( 'NONE', #76746, #91869, #55912 ) ;
#69947=AXIS2_PLACEMENT_3D ( 'NONE', #76376, #18140, #12438 ) ;
#69982=AXIS2_PLACEMENT_3D ( 'NONE', #46457, #23304, #16658 ) ;
#69995=DIRECTION ( 'NONE',  ( -1.000000000000000000, 0.000000000000000000, 0.000000000000000000 ) ) ;
#70039=ORIENTED_EDGE ( 'NONE', *, *, #38462, .F. ) ;
#70050=ORIENTED_EDGE ( 'NONE', *, *, #74984, .F. ) ;
#70084=ORIENTED_EDGE ( 'NONE', *, *, #27513, .T. ) ;
#70090=ADVANCED_FACE ( 'NONE', ( #29348 ), #35039, .T. ) ;
#70114=DIRECTION ( 'NONE',  ( 0.000000000000000000, 0.000000000000000000, -1.000000000000000000 ) ) ;
#70158=CARTESIAN_POINT ( 'NONE',  ( 222.4306832106270804, -142.7221692137691775, -21.50000000000000000 ) ) ;
#70161=VECTOR ( 'NONE', #25346, 1000.000000000000114 ) ;
#70176=VERTEX_POINT ( 'NONE', #13747 ) ;
#70178=CIRCLE ( 'NONE', #33867, 7.999999999999992895 ) ;
#70187=EDGE_LOOP ( 'NONE', ( #6126, #4493, #24628, #17018 ) ) ;
#70190=VECTOR ( 'NONE', #55057, 1000.000000000000000 ) ;
#70195=CARTESIAN_POINT ( 'NONE',  ( 165.2494399300530290, -11.64849832608277325, -3.999999999999998224 ) ) ;
#70238=AXIS2_PLACEMENT_3D ( 'NONE', #3948, #2552, #82995 ) ;
#70242=CARTESIAN_POINT ( 'NONE',  ( 194.7510731661265595, -164.3527196417747689, 21.50000000000000000 ) ) ;
#70244=AXIS2_PLACEMENT_3D ( 'NONE', #90336, #33066, #54369 ) ;
#70256=AXIS2_PLACEMENT_3D ( 'NONE', #75866, #68781, #76346 ) ;
#70263=CARTESIAN_POINT ( 'NONE',  ( 221.8344101925596306, -43.55766379199612004, -22.50000000000000000 ) ) ;
#70271=CIRCLE ( 'NONE', #92955, 1.000000000000000888 ) ;
#70292=EDGE_CURVE ( 'NONE', #67510, #73033, #48831, .T. ) ;
#70302=VERTEX_POINT ( 'NONE', #79070 ) ;
#70418=CARTESIAN_POINT ( 'NONE',  ( 73.43068321062709458, -178.2391364535880882, -4.999999999999990230 ) ) ;
#70432=ORIENTED_EDGE ( 'NONE', *, *, #5214, .F. ) ;
#70438=CARTESIAN_POINT ( 'NONE',  ( 142.6449502718966755, -0.9999999999999991118, 22.50000000000000000 ) ) ;
#70439=CARTESIAN_POINT ( 'NONE',  ( 222.8344101925596306, -44.55766379199611293, -22.08578643762690419 ) ) ;
#70449=VERTEX_POINT ( 'NONE', #80917 ) ;
#70488=FACE_BOUND ( 'NONE', #82906, .T. ) ;
#70526=DIRECTION ( 'NONE',  ( -0.000000000000000000, -0.000000000000000000, 1.000000000000000000 ) ) ;
#70598=LINE ( 'NONE', #19448, #3362 ) ;
#70607=EDGE_CURVE ( 'NONE', #76418, #72836, #53363, .T. ) ;
#70610=DIRECTION ( 'NONE',  ( 0.000000000000000000, 0.000000000000000000, 1.000000000000000000 ) ) ;
#70625=EDGE_CURVE ( 'NONE', #79604, #60489, #52032, .T. ) ;
#70638=ORIENTED_EDGE ( 'NONE', *, *, #16017, .F. ) ;
#70667=CARTESIAN_POINT ( 'NONE',  ( 222.8344101925596306, 7.222594520736746447E-16, 22.08578643762690419 ) ) ;
#70703=CARTESIAN_POINT ( 'NONE',  ( 60.83730532400069535, -250.0090898647485176, -21.50000000000000000 ) ) ;
#70723=EDGE_LOOP ( 'NONE', ( #93661, #16966 ) ) ;
#70761=EDGE_CURVE ( 'NONE', #15223, #90518, #65507, .T. ) ;
#70782=ORIENTED_EDGE ( 'NONE', *, *, #57774, .F. ) ;
#70860=EDGE_LOOP ( 'NONE', ( #15337, #16349, #16385, #54498 ) ) ;
#70936=DIRECTION ( 'NONE',  ( 1.000000000000000000, 0.000000000000000000, 0.000000000000000000 ) ) ;
#70970=VERTEX_POINT ( 'NONE', #11280 ) ;
#70971=CARTESIAN_POINT ( 'NONE',  ( 208.4306832106271088, 42.44233620800392970, 0.000000000000000000 ) ) ;
#70976=ORIENTED_EDGE ( 'NONE', *, *, #31797, .T. ) ;
#71024=ADVANCED_FACE ( 'NONE', ( #92202, #5592, #4179 ), #26424, .T. ) ;
#71048=CARTESIAN_POINT ( 'NONE',  ( -5.802570524182334211, -229.5268262511776527, 22.47499999999998721 ) ) ;
#71052=CIRCLE ( 'NONE', #93671, 8.222204860432944074 ) ;
#71172=CARTESIAN_POINT ( 'NONE',  ( 221.8344101925596306, 15.36528803885690664, 22.50000000000000000 ) ) ;
#71186=ORIENTED_EDGE ( 'NONE', *, *, #6503, .F. ) ;
#71269=EDGE_CURVE ( 'NONE', #67510, #13434, #83231, .T. ) ;
#71359=CARTESIAN_POINT ( 'NONE',  ( 222.8344101925596306, -44.55766379199612004, -21.49999999999998579 ) ) ;
#71451=CIRCLE ( 'NONE', #54789, 4.999999999999990230 ) ;
#71455=FACE_OUTER_BOUND ( 'NONE', #39136, .T. ) ;
#71460=ADVANCED_FACE ( 'NONE', ( #78029 ), #29224, .T. ) ;
#71461=VECTOR ( 'NONE', #2674, 1000.000000000000000 ) ;
#71523=AXIS2_PLACEMENT_3D ( 'NONE', #80793, #74624, #9753 ) ;
#71577=VERTEX_POINT ( 'NONE', #49593 ) ;
#71600=TOROIDAL_SURFACE ( 'NONE', #79095, 8.222204860432958284, 1.000000000000000000 ) ;
#71642=LINE ( 'NONE', #71172, #1348 ) ;
#71663=ORIENTED_EDGE ( 'NONE', *, *, #85914, .F. ) ;
#71691=CARTESIAN_POINT ( 'NONE',  ( 196.7510731661265595, -141.7221692137691775, 21.50000000000000000 ) ) ;
#71697=AXIS2_PLACEMENT_3D ( 'NONE', #50575, #21224, #71911 ) ;
#71721=ORIENTED_EDGE ( 'NONE', *, *, #9205, .T. ) ;
#71878=ADVANCED_FACE ( 'NONE', ( #57190, #43420, #7436 ), #36318, .F. ) ;
#71882=LINE ( 'NONE', #7451, #21845 ) ;
#71890=FACE_OUTER_BOUND ( 'NONE', #24481, .T. ) ;
#71898=CARTESIAN_POINT ( 'NONE',  ( 60.83509176750334291, -250.0104861964972258, 21.50000000000000000 ) ) ;
#71909=DIRECTION ( 'NONE',  ( -1.000000000000000000, 0.000000000000000000, 0.000000000000000000 ) ) ;
#71911=DIRECTION ( 'NONE',  ( -1.000000000000000000, 0.000000000000000000, 0.000000000000000000 ) ) ;
#71924=CARTESIAN_POINT ( 'NONE',  ( 17.06571399127465583, -89.54582641780471874, 21.50000000000000000 ) ) ;
#72030=VECTOR ( 'NONE', #46261, 1000.000000000000114 ) ;
#72058=VERTEX_POINT ( 'NONE', #59975 ) ;
#72074=ADVANCED_FACE ( 'NONE', ( #39078 ), #3562, .F. ) ;
#72112=DIRECTION ( 'NONE',  ( -1.000000000000000000, 0.000000000000000000, 0.000000000000000000 ) ) ;
#72125=VERTEX_POINT ( 'NONE', #52836 ) ;
#72138=EDGE_LOOP ( 'NONE', ( #77767, #51765, #79912, #14666 ) ) ;
#72161=ORIENTED_EDGE ( 'NONE', *, *, #28909, .F. ) ;
#72204=EDGE_CURVE ( 'NONE', #63355, #6488, #2081, .T. ) ;
#72213=DIRECTION ( 'NONE',  ( -0.000000000000000000, -0.000000000000000000, -1.000000000000000000 ) ) ;
#72284=CARTESIAN_POINT ( 'NONE',  ( 139.6925840978351516, -0.9999999999999991118, 22.50000000000000000 ) ) ;
#72369=ORIENTED_EDGE ( 'NONE', *, *, #79409, .F. ) ;
#72421=CARTESIAN_POINT ( 'NONE',  ( 123.4306832106270946, -134.2391364535880882, 0.000000000000000000 ) ) ;
#72472=CARTESIAN_POINT ( 'NONE',  ( 143.6449502718966755, -26.00396092263537540, 21.50000000000000000 ) ) ;
#72584=ORIENTED_EDGE ( 'NONE', *, *, #34074, .F. ) ;
#72658=TOROIDAL_SURFACE ( 'NONE', #4583, 12.40608546931776957, 1.000000000000000000 ) ;
#72664=VECTOR ( 'NONE', #31917, 1000.000000000000000 ) ;
#72818=EDGE_LOOP ( 'NONE', ( #41016, #61106, #17035, #52208 ) ) ;
#72831=DIRECTION ( 'NONE',  ( 1.000000000000000000, 0.000000000000000000, 0.000000000000000000 ) ) ;
#72832=CARTESIAN_POINT ( 'NONE',  ( 60.30377782462291236, -249.1633071459562245, 22.50000000000000000 ) ) ;
#72836=VERTEX_POINT ( 'NONE', #67992 ) ;
#72870=ORIENTED_EDGE ( 'NONE', *, *, #1142, .F. ) ;
#72887=DIRECTION ( 'NONE',  ( -0.000000000000000000, -0.000000000000000000, -1.000000000000000000 ) ) ;
#72942=CARTESIAN_POINT ( 'NONE',  ( 184.7149167944524493, -12.49482340714361506, -6.403442476110241977 ) ) ;
#72991=AXIS2_PLACEMENT_3D ( 'NONE', #48882, #75896, #83931 ) ;
#73018=AXIS2_PLACEMENT_3D ( 'NONE', #81976, #38885, #89536 ) ;
#73023=CARTESIAN_POINT ( 'NONE',  ( 194.5881128153457098, -26.00396092263537540, 21.50000000000000000 ) ) ;
#73033=VERTEX_POINT ( 'NONE', #57082 ) ;
#73071=ORIENTED_EDGE ( 'NONE', *, *, #74867, .T. ) ;
#73123=AXIS2_PLACEMENT_3D ( 'NONE', #65232, #22118, #79872 ) ;
#73131=TOROIDAL_SURFACE ( 'NONE', #54997, 12.40608546931776957, 1.000000000000000000 ) ;
#73133=DIRECTION ( 'NONE',  ( -0.000000000000000000, -0.000000000000000000, 1.000000000000000000 ) ) ;
#73138=CARTESIAN_POINT ( 'NONE',  ( -47.80257052418233599, -229.5268262511776527, 22.50000000000000000 ) ) ;
#73213=PRODUCT ( 'cast Iron C-Frame Chassis', 'cast Iron C-Frame Chassis', '', ( #11814 ) ) ;
#73220=LINE ( 'NONE', #72284, #76470 ) ;
#73275=EDGE_CURVE ( 'NONE', #65497, #72058, #16557, .T. ) ;
#73319=ADVANCED_FACE ( 'NONE', ( #78377 ), #45248, .F. ) ;
#73336=DIRECTION ( 'NONE',  ( 1.000000000000000000, -1.124465274301078034E-16, 0.000000000000000000 ) ) ;
#73376=EDGE_CURVE ( 'NONE', #93680, #30132, #58006, .T. ) ;
#73380=DIRECTION ( 'NONE',  ( 0.000000000000000000, -1.000000000000000000, 0.000000000000000000 ) ) ;
#73438=EDGE_LOOP ( 'NONE', ( #5558, #62957, #43225, #75529 ) ) ;
#73480=FACE_OUTER_BOUND ( 'NONE', #19925, .T. ) ;
#73525=DIRECTION ( 'NONE',  ( 1.000000000000000000, 0.000000000000000000, 0.000000000000000000 ) ) ;
#73570=DIRECTION ( 'NONE',  ( -1.000000000000000000, 0.000000000000000000, 0.000000000000000000 ) ) ;
#73573=EDGE_CURVE ( 'NONE', #9702, #14431, #2092, .T. ) ;
#73628=ADVANCED_FACE ( 'NONE', ( #66498 ), #69481, .F. ) ;
#73682=CARTESIAN_POINT ( 'NONE',  ( 184.7149167944524493, -12.49482340714361506, 10.00000000000000000 ) ) ;
#73711=DIRECTION ( 'NONE',  ( -0.8043439146810466012, -0.5941640067486159138, 0.000000000000000000 ) ) ;
#73765=CARTESIAN_POINT ( 'NONE',  ( 2.197429475817664013, -229.5268262511776527, 22.47499999999998721 ) ) ;
#73898=EDGE_CURVE ( 'NONE', #77341, #25970, #71052, .T. ) ;
#73951=ORIENTED_EDGE ( 'NONE', *, *, #30285, .F. ) ;
#73959=EDGE_CURVE ( 'NONE', #40992, #60489, #43782, .T. ) ;
#74017=DIRECTION ( 'NONE',  ( 1.000000000000000000, 0.000000000000000000, 0.000000000000000000 ) ) ;
#74037=DIRECTION ( 'NONE',  ( -1.000000000000000000, 0.000000000000000000, 0.000000000000000000 ) ) ;
#74125=DIRECTION ( 'NONE',  ( 0.000000000000000000, 0.000000000000000000, 1.000000000000000000 ) ) ;
#74128=AXIS2_PLACEMENT_3D ( 'NONE', #82120, #89674, #17738 ) ;
#74170=LINE ( 'NONE', #65716, #62263 ) ;
#74194=CIRCLE ( 'NONE', #12671, 1.000000000000000888 ) ;
#74197=EDGE_LOOP ( 'NONE', ( #92389, #82694, #82950, #67335 ) ) ;
#74242=DIRECTION ( 'NONE',  ( 1.000000000000000000, 0.000000000000000000, 0.000000000000000000 ) ) ;
#74285=CARTESIAN_POINT ( 'NONE',  ( 123.4306832106270946, -134.2391364535880882, 5.024999999999987921 ) ) ;
#74306=ORIENTED_EDGE ( 'NONE', *, *, #39352, .T. ) ;
#74335=CIRCLE ( 'NONE', #83377, 1.000000000000000888 ) ;
#74347=VERTEX_POINT ( 'NONE', #10110 ) ;
#74365=ORIENTED_EDGE ( 'NONE', *, *, #5214, .T. ) ;
#74411=DIRECTION ( 'NONE',  ( -0.000000000000000000, 1.000000000000000000, -0.000000000000000000 ) ) ;
#74414=CARTESIAN_POINT ( 'NONE',  ( 169.2494399300530290, -11.64849832608277325, -3.999999999999998224 ) ) ;
#74473=VECTOR ( 'NONE', #63815, 1000.000000000000000 ) ;
#74479=ORIENTED_EDGE ( 'NONE', *, *, #46910, .F. ) ;
#74480=CARTESIAN_POINT ( 'NONE',  ( 222.4306832106270804, -141.7221692137691775, -21.50000000000000000 ) ) ;
#74501=DIRECTION ( 'NONE',  ( -0.000000000000000000, -0.000000000000000000, 1.000000000000000000 ) ) ;
#74615=CARTESIAN_POINT ( 'NONE',  ( -23.40286736638519471, -122.5496321078137356, -21.50000000000000000 ) ) ;
#74624=DIRECTION ( 'NONE',  ( -1.000000000000000000, 0.000000000000000000, 0.000000000000000000 ) ) ;
#74650=DIRECTION ( 'NONE',  ( -0.000000000000000000, -0.000000000000000000, -1.000000000000000000 ) ) ;
#74658=CARTESIAN_POINT ( 'NONE',  ( 165.2494399300530290, -11.64849832608277325, 10.00000000000000000 ) ) ;
#74661=DIRECTION ( 'NONE',  ( -1.000000000000000000, 0.000000000000000000, 0.000000000000000000 ) ) ;
#74689=CARTESIAN_POINT ( 'NONE',  ( 60.29495240252359878, -249.1689065933675238, -22.50000000000000000 ) ) ;
#74706=VERTEX_POINT ( 'NONE', #3479 ) ;
#74732=CARTESIAN_POINT ( 'NONE',  ( 208.4306832106271088, -44.55766379199612004, 0.000000000000000000 ) ) ;
#74739=ADVANCED_FACE ( 'NONE', ( #91511 ), #37759, .F. ) ;
#74753=DIRECTION ( 'NONE',  ( -0.000000000000000000, -0.000000000000000000, 1.000000000000000000 ) ) ;
#74768=DIRECTION ( 'NONE',  ( -1.000000000000000000, 0.000000000000000000, 0.000000000000000000 ) ) ;
#74770=DIRECTION ( 'NONE',  ( 0.000000000000000000, 0.000000000000000000, -1.000000000000000000 ) ) ;
#74797=CARTESIAN_POINT ( 'NONE',  ( -23.40286736638519471, -134.2391364535880598, -21.49999999999998579 ) ) ;
#74830=CIRCLE ( 'NONE', #53673, 203.9779373800640485 ) ;
#74849=VECTOR ( 'NONE', #62873, 1000.000000000000000 ) ;
#74867=EDGE_CURVE ( 'NONE', #33292, #76418, #20964, .T. ) ;
#74900=DIRECTION ( 'NONE',  ( -0.000000000000000000, 1.000000000000000000, -0.000000000000000000 ) ) ;
#74908=VECTOR ( 'NONE', #82735, 1000.000000000000000 ) ;
#74919=FACE_OUTER_BOUND ( 'NONE', #24004, .T. ) ;
#74954=DIRECTION ( 'NONE',  ( -0.8571673007021122226, 1.049727191138618696E-16, 0.5150380749100541555 ) ) ;
#74982=CARTESIAN_POINT ( 'NONE',  ( 123.4306832106270946, -178.2391364535880882, 4.999999999999990230 ) ) ;
#74984=EDGE_CURVE ( 'NONE', #43035, #22436, #86100, .T. ) ;
#74989=DIRECTION ( 'NONE',  ( 0.000000000000000000, 0.000000000000000000, 1.000000000000000000 ) ) ;
#75002=DIRECTION ( 'NONE',  ( -1.000000000000000000, 0.000000000000000000, 0.000000000000000000 ) ) ;
#75129=CARTESIAN_POINT ( 'NONE',  ( 139.6925840978351516, 15.36528803885690664, 21.50000000000000000 ) ) ;
#75155=DIRECTION ( 'NONE',  ( -1.000000000000000000, 0.000000000000000000, 0.000000000000000000 ) ) ;
#75169=ORIENTED_EDGE ( 'NONE', *, *, #67180, .T. ) ;
#75213=EDGE_CURVE ( 'NONE', #74347, #87117, #35648, .T. ) ;
#75225=CARTESIAN_POINT ( 'NONE',  ( 17.06571399127465583, -89.54582641780471874, 22.50000000000000000 ) ) ;
#75251=CARTESIAN_POINT ( 'NONE',  ( -56.02477538461528184, -229.5268262511776527, 21.50000000000000000 ) ) ;
#75254=DIRECTION ( 'NONE',  ( 1.000000000000000000, 0.000000000000000000, 0.000000000000000000 ) ) ;
#75339=FACE_OUTER_BOUND ( 'NONE', #17996, .T. ) ;
#75372=DIRECTION ( 'NONE',  ( 0.000000000000000000, 0.000000000000000000, 1.000000000000000000 ) ) ;
#75529=ORIENTED_EDGE ( 'NONE', *, *, #85679, .F. ) ;
#75574=DIRECTION ( 'NONE',  ( 0.000000000000000000, 0.000000000000000000, 1.000000000000000000 ) ) ;
#75598=ORIENTED_EDGE ( 'NONE', *, *, #43751, .T. ) ;
#75656=VERTEX_POINT ( 'NONE', #17997 ) ;
#75708=VERTEX_POINT ( 'NONE', #46850 ) ;
#75740=EDGE_CURVE ( 'NONE', #56465, #18301, #92241, .T. ) ;
#75758=DIRECTION ( 'NONE',  ( -0.000000000000000000, 1.000000000000000000, -0.000000000000000000 ) ) ;
#75798=DIRECTION ( 'NONE',  ( 0.000000000000000000, 0.000000000000000000, 1.000000000000000000 ) ) ;
#75814=ORIENTED_EDGE ( 'NONE', *, *, #22374, .F. ) ;
#75846=VERTEX_POINT ( 'NONE', #93232 ) ;
#75866=CARTESIAN_POINT ( 'NONE',  ( 61.37083282337847123, -250.8548725835408391, -21.49999999999999289 ) ) ;
#75871=ORIENTED_EDGE ( 'NONE', *, *, #72204, .T. ) ;
#75890=DIRECTION ( 'NONE',  ( -0.5941640067486292365, -0.8043439146810368312, 0.000000000000000000 ) ) ;
#75896=DIRECTION ( 'NONE',  ( -0.000000000000000000, -0.000000000000000000, 1.000000000000000000 ) ) ;
#75932=CARTESIAN_POINT ( 'NONE',  ( -36.09237171215954021, -122.5496321078137356, -21.50000000000000000 ) ) ;
#75934=ORIENTED_EDGE ( 'NONE', *, *, #79929, .F. ) ;
#75936=DIRECTION ( 'NONE',  ( 0.8457827187922973833, 0.5335274993777826547, 0.000000000000000000 ) ) ;
#75952=AXIS2_PLACEMENT_3D ( 'NONE', #73682, #31525, #17324 ) ;
#75954=AXIS2_PLACEMENT_3D ( 'NONE', #78514, #13651, #86056 ) ;
#75959=AXIS2_PLACEMENT_3D ( 'NONE', #11165, #63264, #92095 ) ;
#76021=CIRCLE ( 'NONE', #77586, 1.000000000000000888 ) ;
#76029=CIRCLE ( 'NONE', #50283, 1.000000000000000888 ) ;
#76054=DIRECTION ( 'NONE',  ( -1.000000000000000000, 0.000000000000000000, 0.000000000000000000 ) ) ;
#76057=CIRCLE ( 'NONE', #69982, 1.000000000000000888 ) ;
#76071=CARTESIAN_POINT ( 'NONE',  ( 194.7510731661265595, -164.3527196417747689, -21.50000000000000000 ) ) ;
#76083=CARTESIAN_POINT ( 'NONE',  ( 139.6925840978351516, 15.36528803885690664, -22.50000000000000000 ) ) ;
#76096=LINE ( 'NONE', #81780, #35724 ) ;
#76100=ORIENTED_EDGE ( 'NONE', *, *, #40423, .T. ) ;
#76147=CARTESIAN_POINT ( 'NONE',  ( 222.4306832106270804, 15.36528803885690664, 22.50000000000000000 ) ) ;
#76183=ORIENTED_EDGE ( 'NONE', *, *, #2076, .T. ) ;
#76232=CARTESIAN_POINT ( 'NONE',  ( 223.4306832106270804, -135.2391364535880882, -22.50000000000000000 ) ) ;
#76237=CIRCLE ( 'NONE', #6707, 2.000000000000001776 ) ;
#76268=EDGE_CURVE ( 'NONE', #5915, #70302, #14652, .T. ) ;
#76312=FACE_BOUND ( 'NONE', #17529, .T. ) ;
#76327=ORIENTED_EDGE ( 'NONE', *, *, #5345, .F. ) ;
#76346=DIRECTION ( 'NONE',  ( -1.000000000000000000, 6.661338147750933184E-13, 0.000000000000000000 ) ) ;
#76360=DIRECTION ( 'NONE',  ( -0.000000000000000000, -0.000000000000000000, 1.000000000000000000 ) ) ;
#76376=CARTESIAN_POINT ( 'NONE',  ( -22.78264641048746597, -118.9815703160634541, 21.50000000000000000 ) ) ;
#76386=EDGE_CURVE ( 'NONE', #19742, #4433, #39660, .T. ) ;
#76390=CARTESIAN_POINT ( 'NONE',  ( 184.7149167944524493, -12.49482340714361506, -3.999999999999998224 ) ) ;
#76401=DIRECTION ( 'NONE',  ( 0.000000000000000000, 0.000000000000000000, -1.000000000000000000 ) ) ;
#76418=VERTEX_POINT ( 'NONE', #42140 ) ;
#76470=VECTOR ( 'NONE', #14534, 1000.000000000000000 ) ;
#76557=CYLINDRICAL_SURFACE ( 'NONE', #6292, 1.000000000000000888 ) ;
#76596=DIRECTION ( 'NONE',  ( -0.000000000000000000, -0.000000000000000000, -1.000000000000000000 ) ) ;
#76600=ORIENTED_EDGE ( 'NONE', *, *, #2175, .T. ) ;
#76671=FACE_OUTER_BOUND ( 'NONE', #30013, .T. ) ;
#76692=VERTEX_POINT ( 'NONE', #49728 ) ;
#76732=CARTESIAN_POINT ( 'NONE',  ( 194.7510731661265595, -164.3527196417747689, 21.50000000000000000 ) ) ;
#76744=DIRECTION ( 'NONE',  ( -0.000000000000000000, -1.000000000000000000, -0.000000000000000000 ) ) ;
#76746=CARTESIAN_POINT ( 'NONE',  ( -36.09237171215955442, -55.96374926131388605, -21.50000000000000000 ) ) ;
#76828=ORIENTED_EDGE ( 'NONE', *, *, #87492, .T. ) ;
#76916=ADVANCED_FACE ( 'NONE', ( #11646, #40493 ), #33417, .F. ) ;
#76931=ORIENTED_EDGE ( 'NONE', *, *, #86325, .T. ) ;
#76937=ORIENTED_EDGE ( 'NONE', *, *, #4015, .F. ) ;
#77058=CARTESIAN_POINT ( 'NONE',  ( -23.40286736638519471, -122.5496321078137356, -22.50000000000000000 ) ) ;
#77089=EDGE_CURVE ( 'NONE', #72836, #77341, #57538, .T. ) ;
#77134=ORIENTED_EDGE ( 'NONE', *, *, #34031, .F. ) ;
#77158=ADVANCED_FACE ( 'NONE', ( #29610 ), #8730, .T. ) ;
#77241=CARTESIAN_POINT ( 'NONE',  ( 194.5881128153457098, 0.000000000000000000, -47.19625681453479871 ) ) ;
#77294=VERTEX_POINT ( 'NONE', #22481 ) ;
#77301=FACE_OUTER_BOUND ( 'NONE', #89372, .T. ) ;
#77341=VERTEX_POINT ( 'NONE', #51816 ) ;
#77348=CYLINDRICAL_SURFACE ( 'NONE', #6572, 1.000000000000002887 ) ;
#77380=ORIENTED_EDGE ( 'NONE', *, *, #16494, .T. ) ;
#77485=ORIENTED_EDGE ( 'NONE', *, *, #32100, .T. ) ;
#77496=DIRECTION ( 'NONE',  ( 1.049727191138620051E-16, 0.5150380749100522682, -0.8571673007021134438 ) ) ;
#77531=ORIENTED_EDGE ( 'NONE', *, *, #79929, .T. ) ;
#77586=AXIS2_PLACEMENT_3D ( 'NONE', #74480, #74017, #81572 ) ;
#77679=DIRECTION ( 'NONE',  ( 0.7071067811864494290, 0.000000000000000000, 0.7071067811866457165 ) ) ;
#77701=EDGE_CURVE ( 'NONE', #28617, #6151, #24820, .T. ) ;
#77704=ORIENTED_EDGE ( 'NONE', *, *, #10535, .T. ) ;
#77747=CIRCLE ( 'NONE', #36924, 1.000000000000000888 ) ;
#77753=EDGE_CURVE ( 'NONE', #13434, #76692, #66975, .T. ) ;
#77767=ORIENTED_EDGE ( 'NONE', *, *, #71269, .F. ) ;
#77822=CARTESIAN_POINT ( 'NONE',  ( 169.2744399300530347, -11.64849832608277325, 10.00000000000000000 ) ) ;
#77829=CIRCLE ( 'NONE', #29436, 11.40608546931776779 ) ;
#77831=EDGE_CURVE ( 'NONE', #12908, #37793, #46933, .T. ) ;
#77875=ADVANCED_FACE ( 'NONE', ( #60350 ), #54156, .F. ) ;
#77891=ORIENTED_EDGE ( 'NONE', *, *, #14175, .F. ) ;
#77901=AXIS2_PLACEMENT_3D ( 'NONE', #68170, #33113, #68642 ) ;
#77907=AXIS2_PLACEMENT_3D ( 'NONE', #57173, #22101, #93583 ) ;
#77967=CONICAL_SURFACE ( 'NONE', #11506, 4.025000000000000355, 0.7853981633973095011 ) ;
#77969=EDGE_LOOP ( 'NONE', ( #7088, #62606, #39290, #56302 ) ) ;
#77986=VERTEX_POINT ( 'NONE', #10594 ) ;
#78013=VERTEX_POINT ( 'NONE', #77822 ) ;
#78029=FACE_OUTER_BOUND ( 'NONE', #56104, .T. ) ;
#78090=CARTESIAN_POINT ( 'NONE',  ( 165.2494399300530290, -11.64849832608277325, 10.00000000000000000 ) ) ;
#78144=DIRECTION ( 'NONE',  ( -0.000000000000000000, -1.000000000000000000, -0.000000000000000000 ) ) ;
#78145=DIRECTION ( 'NONE',  ( 1.000000000000000000, 0.000000000000000000, 0.000000000000000000 ) ) ;
#78205=ORIENTED_EDGE ( 'NONE', *, *, #90641, .F. ) ;
#78272=DIRECTION ( 'NONE',  ( -0.000000000000000000, -0.000000000000000000, 1.000000000000000000 ) ) ;
#78289=ORIENTED_EDGE ( 'NONE', *, *, #5090, .F. ) ;
#78292=CARTESIAN_POINT ( 'NONE',  ( 221.8344101925596306, 15.36528803885690664, 21.50000000000000000 ) ) ;
#78324=EDGE_LOOP ( 'NONE', ( #6970, #66246, #7277, #26151 ) ) ;
#78350=ORIENTED_EDGE ( 'NONE', *, *, #87501, .F. ) ;
#78352=ADVANCED_FACE ( 'NONE', ( #19574 ), #83250, .F. ) ;
#78353=ORIENTED_EDGE ( 'NONE', *, *, #69069, .F. ) ;
#78377=FACE_OUTER_BOUND ( 'NONE', #37610, .T. ) ;
#78431=VERTEX_POINT ( 'NONE', #70263 ) ;
#78462=CYLINDRICAL_SURFACE ( 'NONE', #9500, 15.36528803885689420 ) ;
#78468=DIRECTION ( 'NONE',  ( -1.000000000000000000, -0.000000000000000000, -0.000000000000000000 ) ) ;
#78469=DIRECTION ( 'NONE',  ( -0.000000000000000000, -0.000000000000000000, -1.000000000000000000 ) ) ;
#78512=ADVANCED_FACE ( 'NONE', ( #56040, #83970 ), #33311, .F. ) ;
#78514=CARTESIAN_POINT ( 'NONE',  ( -147.0026986695707762, 31.65052214425332622, -21.50000000000000000 ) ) ;
#78543=FACE_OUTER_BOUND ( 'NONE', #60076, .T. ) ;
#78552=FACE_OUTER_BOUND ( 'NONE', #21258, .T. ) ;
#78615=CARTESIAN_POINT ( 'NONE',  ( 208.4306832106271088, -134.2391364535880882, 0.000000000000000000 ) ) ;
#78654=FACE_OUTER_BOUND ( 'NONE', #27776, .T. ) ;
#78655=CARTESIAN_POINT ( 'NONE',  ( 73.43068321062709458, -178.2391364535880882, 4.999999999999990230 ) ) ;
#78683=DIRECTION ( 'NONE',  ( 1.000000000000000000, 0.000000000000000000, 0.000000000000000000 ) ) ;
#78715=ORIENTED_EDGE ( 'NONE', *, *, #39228, .T. ) ;
#78728=CARTESIAN_POINT ( 'NONE',  ( -55.80257052418232888, -229.5268262511776527, 22.50000000000000000 ) ) ;
#78752=ORIENTED_EDGE ( 'NONE', *, *, #90146, .F. ) ;
#78811=ADVANCED_FACE ( 'NONE', ( #35185 ), #14824, .F. ) ;
#78861=ADVANCED_FACE ( 'NONE', ( #42277 ), #87681, .T. ) ;
#78869=EDGE_CURVE ( 'NONE', #783, #15111, #65037, .T. ) ;
#78883=TOROIDAL_SURFACE ( 'NONE', #35078, 2.000000000000000000, 1.000000000000000000 ) ;
#78886=ORIENTED_EDGE ( 'NONE', *, *, #24174, .T. ) ;
#78925=DIRECTION ( 'NONE',  ( 1.000000000000000000, -0.000000000000000000, 0.000000000000000000 ) ) ;
#78945=DIRECTION ( 'NONE',  ( 0.000000000000000000, 0.000000000000000000, 1.000000000000000000 ) ) ;
#78960=CARTESIAN_POINT ( 'NONE',  ( 73.43068321062709458, -178.2391364535880882, 4.999999999999990230 ) ) ;
#78969=CARTESIAN_POINT ( 'NONE',  ( 60.29495240252358457, -249.1689065933674954, -21.50000000000000000 ) ) ;
#79014=DIRECTION ( 'NONE',  ( 1.000000000000000000, 0.000000000000000000, 0.000000000000000000 ) ) ;
#79027=ORIENTED_EDGE ( 'NONE', *, *, #84489, .T. ) ;
#79070=CARTESIAN_POINT ( 'NONE',  ( -147.8070425842518034, -211.3363389866113664, -21.49999999999998579 ) ) ;
#79086=CIRCLE ( 'NONE', #91130, 4.000000000000003553 ) ;
#79095=AXIS2_PLACEMENT_3D ( 'NONE', #82199, #89281, #2675 ) ;
#79147=ORIENTED_EDGE ( 'NONE', *, *, #76386, .F. ) ;
#79310=AXIS2_PLACEMENT_3D ( 'NONE', #50546, #79443, #70936 ) ;
#79317=DIRECTION ( 'NONE',  ( -0.000000000000000000, -0.000000000000000000, 1.000000000000000000 ) ) ;
#79322=DIRECTION ( 'NONE',  ( -0.000000000000000000, 1.000000000000000000, -0.000000000000000000 ) ) ;
#79342=DIRECTION ( 'NONE',  ( -1.000000000000000000, 0.000000000000000000, 0.000000000000000000 ) ) ;
#79407=CARTESIAN_POINT ( 'NONE',  ( 143.6449502718966755, 0.000000000000000000, 21.50000000000000000 ) ) ;
#79409=EDGE_CURVE ( 'NONE', #29328, #41863, #440, .T. ) ;
#79416=EDGE_CURVE ( 'NONE', #7995, #63355, #17132, .T. ) ;
#79441=FACE_OUTER_BOUND ( 'NONE', #56591, .T. ) ;
#79443=DIRECTION ( 'NONE',  ( -0.000000000000000000, -0.000000000000000000, 1.000000000000000000 ) ) ;
#79493=DIRECTION ( 'NONE',  ( 0.000000000000000000, 0.000000000000000000, 1.000000000000000000 ) ) ;
#79494=FACE_OUTER_BOUND ( 'NONE', #60534, .T. ) ;
#79504=EDGE_LOOP ( 'NONE', ( #65039, #55876, #29734, #64968 ) ) ;
#79552=DIRECTION ( 'NONE',  ( -0.000000000000000000, 1.000000000000000000, -0.000000000000000000 ) ) ;
#79581=EDGE_CURVE ( 'NONE', #6151, #59355, #76057, .T. ) ;
#79593=CYLINDRICAL_SURFACE ( 'NONE', #55702, 1.000000000000000888 ) ;
#79604=VERTEX_POINT ( 'NONE', #74414 ) ;
#79612=ORIENTED_EDGE ( 'NONE', *, *, #2190, .T. ) ;
#79631=ORIENTED_EDGE ( 'NONE', *, *, #61955, .F. ) ;
#79666=DIRECTION ( 'NONE',  ( 0.000000000000000000, 1.000000000000000000, 0.000000000000000000 ) ) ;
#79714=VERTEX_POINT ( 'NONE', #66857 ) ;
#79717=ORIENTED_EDGE ( 'NONE', *, *, #92592, .F. ) ;
#79770=DIRECTION ( 'NONE',  ( -1.000000000000000000, 0.000000000000000000, 0.000000000000000000 ) ) ;
#79787=DIRECTION ( 'NONE',  ( 1.000000000000000000, 0.000000000000000000, 0.000000000000000000 ) ) ;
#79842=ORIENTED_EDGE ( 'NONE', *, *, #89540, .T. ) ;
#79872=DIRECTION ( 'NONE',  ( -1.000000000000000000, 0.000000000000000000, 0.000000000000000000 ) ) ;
#79898=CYLINDRICAL_SURFACE ( 'NONE', #9433, 1.000000000000000888 ) ;
#79912=ORIENTED_EDGE ( 'NONE', *, *, #86325, .F. ) ;
#79925=LINE ( 'NONE', #22170, #65251 ) ;
#79929=EDGE_CURVE ( 'NONE', #40890, #60407, #6525, .T. ) ;
#79936=CARTESIAN_POINT ( 'NONE',  ( 139.6925840978351516, 0.000000000000000000, 21.50000000000000000 ) ) ;
#79974=CARTESIAN_POINT ( 'NONE',  ( 123.4306832106270946, -134.2641364535880939, -4.999999999999990230 ) ) ;
#79978=EDGE_CURVE ( 'NONE', #90108, #51697, #3465, .T. ) ;
#80042=ADVANCED_FACE ( 'NONE', ( #63524 ), #1974, .T. ) ;
#80245=CARTESIAN_POINT ( 'NONE',  ( 222.8344101925596306, -0.9999999999999997780, -21.50000000000000000 ) ) ;
#80248=ADVANCED_FACE ( 'NONE', ( #55926 ), #11424, .F. ) ;
#80294=CIRCLE ( 'NONE', #92372, 5.025000000000002132 ) ;
#80305=EDGE_CURVE ( 'NONE', #21234, #5915, #48804, .T. ) ;
#80313=EDGE_LOOP ( 'NONE', ( #91809, #33250, #6036, #56800 ) ) ;
#80342=DIRECTION ( 'NONE',  ( 0.000000000000000000, 0.000000000000000000, 1.000000000000000000 ) ) ;
#80390=DIRECTION ( 'NONE',  ( -1.000000000000000000, 0.000000000000000000, 0.000000000000000000 ) ) ;
#80494=CARTESIAN_POINT ( 'NONE',  ( 184.7149167944524493, -12.49482340714361506, 10.00000000000000000 ) ) ;
#80496=LINE ( 'NONE', #31715, #49676 ) ;
#80515=ORIENTED_EDGE ( 'NONE', *, *, #37424, .T. ) ;
#80522=DIRECTION ( 'NONE',  ( 0.000000000000000000, 0.000000000000000000, 1.000000000000000000 ) ) ;
#80535=CARTESIAN_POINT ( 'NONE',  ( 73.43068321062709458, -134.2391364535880598, 5.025000000000002132 ) ) ;
#80551=TOROIDAL_SURFACE ( 'NONE', #4936, 12.68950434577434372, 1.000000000000000000 ) ;
#80600=VECTOR ( 'NONE', #69050, 1000.000000000000000 ) ;
#80635=ORIENTED_EDGE ( 'NONE', *, *, #44097, .T. ) ;
#80685=CARTESIAN_POINT ( 'NONE',  ( 165.2494399300530290, -11.64849832608277325, 9.974999999999996092 ) ) ;
#80705=AXIS2_PLACEMENT_3D ( 'NONE', #78969, #64800, #65254 ) ;
#80753=CIRCLE ( 'NONE', #83781, 4.000000000000003553 ) ;
#80781=AXIS2_PLACEMENT_3D ( 'NONE', #4800, #26584, #5293 ) ;
#80793=CARTESIAN_POINT ( 'NONE',  ( 223.4306832106270804, -147.4436952405746979, 22.50000000000000000 ) ) ;
#80798=DIRECTION ( 'NONE',  ( 0.000000000000000000, 0.000000000000000000, -1.000000000000000000 ) ) ;
#80814=LINE ( 'NONE', #32017, #59505 ) ;
#80835=EDGE_CURVE ( 'NONE', #75656, #19742, #29385, .T. ) ;
#80838=EDGE_LOOP ( 'NONE', ( #31376, #67607, #83735, #84829 ) ) ;
#80894=DIRECTION ( 'NONE',  ( 0.000000000000000000, 0.000000000000000000, -1.000000000000000000 ) ) ;
#80917=CARTESIAN_POINT ( 'NONE',  ( 195.7510731661265595, -143.7221692137691775, -21.50000000000000000 ) ) ;
#80951=EDGE_CURVE ( 'NONE', #14431, #17995, #87515, .T. ) ;
#80967=ORIENTED_EDGE ( 'NONE', *, *, #77089, .T. ) ;
#80992=ORIENTED_EDGE ( 'NONE', *, *, #48158, .T. ) ;
#81010=DIRECTION ( 'NONE',  ( 0.000000000000000000, 1.000000000000000000, 0.000000000000000000 ) ) ;
#81031=DIRECTION ( 'NONE',  ( 0.000000000000000000, 0.000000000000000000, -1.000000000000000000 ) ) ;
#81046=DIRECTION ( 'NONE',  ( 0.000000000000000000, 0.000000000000000000, -1.000000000000000000 ) ) ;
#81076=CYLINDRICAL_SURFACE ( 'NONE', #7694, 204.9779373800640485 ) ;
#81263=LINE ( 'NONE', #31553, #71461 ) ;
#81338=DIRECTION ( 'NONE',  ( 0.000000000000000000, 1.000000000000000000, 0.000000000000000000 ) ) ;
#81352=EDGE_LOOP ( 'NONE', ( #72369, #84728 ) ) ;
#81407=CARTESIAN_POINT ( 'NONE',  ( 195.5881128153457098, -0.9999999999999991118, 22.50000000000000000 ) ) ;
#81442=EDGE_LOOP ( 'NONE', ( #28623, #88570, #74365 ) ) ;
#81508=CARTESIAN_POINT ( 'NONE',  ( 123.4306832106270946, -134.2391364535880882, 0.000000000000000000 ) ) ;
#81523=LINE ( 'NONE', #52191, #23337 ) ;
#81524=DIRECTION ( 'NONE',  ( -0.000000000000000000, -0.000000000000000000, -1.000000000000000000 ) ) ;
#81526=CARTESIAN_POINT ( 'NONE',  ( 142.6449502718966755, 15.36528803885690664, 22.50000000000000000 ) ) ;
#81572=DIRECTION ( 'NONE',  ( 0.000000000000000000, 0.000000000000000000, -1.000000000000000000 ) ) ;
#81577=ORIENTED_EDGE ( 'NONE', *, *, #80835, .T. ) ;
#81628=DIRECTION ( 'NONE',  ( -0.000000000000000000, -0.000000000000000000, -1.000000000000000000 ) ) ;
#81693=FACE_OUTER_BOUND ( 'NONE', #41869, .T. ) ;
#81742=FACE_OUTER_BOUND ( 'NONE', #21373, .T. ) ;
#81756=EDGE_LOOP ( 'NONE', ( #17539, #28595, #16015, #63113 ) ) ;
#81769=VERTEX_POINT ( 'NONE', #24118 ) ;
#81780=CARTESIAN_POINT ( 'NONE',  ( 196.7510731661265595, -142.7221692137691775, -22.50000000000000000 ) ) ;
#81803=DIRECTION ( 'NONE',  ( -0.000000000000000000, 0.000000000000000000, 1.000000000000000000 ) ) ;
#81804=LINE ( 'NONE', #88450, #12499 ) ;
#81868=ORIENTED_EDGE ( 'NONE', *, *, #59688, .F. ) ;
#81872=CARTESIAN_POINT ( 'NONE',  ( 194.5881128153456814, 6.505213034913026604E-16, 22.08578643762690419 ) ) ;
#81880=ORIENTED_EDGE ( 'NONE', *, *, #67502, .F. ) ;
#81899=EDGE_LOOP ( 'NONE', ( #39593, #44380 ) ) ;
#81976=CARTESIAN_POINT ( 'NONE',  ( 123.4306832106270946, -134.2391364535880882, 0.000000000000000000 ) ) ;
#81991=EDGE_CURVE ( 'NONE', #44672, #44867, #7612, .T. ) ;
#81994=LINE ( 'NONE', #23782, #22831 ) ;
#82029=VECTOR ( 'NONE', #37756, 1000.000000000000000 ) ;
#82034=EDGE_LOOP ( 'NONE', ( #84213, #52013, #56790, #52695 ) ) ;
#82042=EDGE_LOOP ( 'NONE', ( #37293, #36888, #7473, #10164 ) ) ;
#82047=VERTEX_POINT ( 'NONE', #74797 ) ;
#82064=CARTESIAN_POINT ( 'NONE',  ( 208.4306832106271088, -142.7221692137691775, 0.000000000000000000 ) ) ;
#82077=DIRECTION ( 'NONE',  ( -0.000000000000000000, -0.000000000000000000, -1.000000000000000000 ) ) ;
#82092=TOROIDAL_SURFACE ( 'NONE', #1948, 8.222204860432942297, 1.000000000000000000 ) ;
#82099=CARTESIAN_POINT ( 'NONE',  ( -23.40286736638519471, -134.2391364535880598, 22.50000000000000000 ) ) ;
#82103=VECTOR ( 'NONE', #45632, 1000.000000000000000 ) ;
#82120=CARTESIAN_POINT ( 'NONE',  ( 17.06571399127465583, -89.54582641780471874, 22.50000000000000000 ) ) ;
#82139=ADVANCED_FACE ( 'NONE', ( #53473 ), #17500, .F. ) ;
#82162=CIRCLE ( 'NONE', #20202, 1.000000000000007105 ) ;
#82199=CARTESIAN_POINT ( 'NONE',  ( 2.197429475817664013, -229.5268262511776527, 21.50000000000000000 ) ) ;
#82249=AXIS2_PLACEMENT_3D ( 'NONE', #37368, #25042, #24093 ) ;
#82282=CARTESIAN_POINT ( 'NONE',  ( 222.4306832106270804, -141.7221692137691775, -21.50000000000000000 ) ) ;
#82291=DIRECTION ( 'NONE',  ( -1.000000000000000000, 0.000000000000000000, 0.000000000000000000 ) ) ;
#82296=CARTESIAN_POINT ( 'NONE',  ( 208.4306832106271088, 42.44233620800392970, 0.000000000000000000 ) ) ;
#82386=EDGE_CURVE ( 'NONE', #783, #30831, #11096, .T. ) ;
#82409=CARTESIAN_POINT ( 'NONE',  ( 139.6925840978351516, -0.9999999999999991118, 21.50000000000000000 ) ) ;
#82418=CARTESIAN_POINT ( 'NONE',  ( 194.7510731661265595, 15.36528803885690664, 21.50000000000000000 ) ) ;
#82488=VERTEX_POINT ( 'NONE', #91774 ) ;
#82496=DIRECTION ( 'NONE',  ( -0.000000000000000000, 1.000000000000000000, -0.000000000000000000 ) ) ;
#82544=EDGE_CURVE ( 'NONE', #26494, #18590, #83681, .T. ) ;
#82621=ORIENTED_EDGE ( 'NONE', *, *, #64250, .F. ) ;
#82669=DIRECTION ( 'NONE',  ( -0.000000000000000000, -0.000000000000000000, -1.000000000000000000 ) ) ;
#82694=ORIENTED_EDGE ( 'NONE', *, *, #85679, .T. ) ;
#82697=FACE_OUTER_BOUND ( 'NONE', #8091, .T. ) ;
#82735=DIRECTION ( 'NONE',  ( 1.124465274301078281E-16, 1.000000000000000000, -0.000000000000000000 ) ) ;
#82738=DIRECTION ( 'NONE',  ( 1.000000000000000000, 0.000000000000000000, 0.000000000000000000 ) ) ;
#82782=DIRECTION ( 'NONE',  ( -1.000000000000000000, 0.000000000000000000, 0.000000000000000000 ) ) ;
#82882=CYLINDRICAL_SURFACE ( 'NONE', #64053, 7.500000000000007105 ) ;
#82889=CYLINDRICAL_SURFACE ( 'NONE', #54719, 1.000000000000000888 ) ;
#82902=ADVANCED_FACE ( 'NONE', ( #13668 ), #56286, .F. ) ;
#82906=EDGE_LOOP ( 'NONE', ( #67125, #44668 ) ) ;
#82950=ORIENTED_EDGE ( 'NONE', *, *, #77701, .F. ) ;
#82995=DIRECTION ( 'NONE',  ( 1.000000000000000000, 0.000000000000000000, 0.000000000000000000 ) ) ;
#83009=FACE_OUTER_BOUND ( 'NONE', #1918, .T. ) ;
#83025=DIRECTION ( 'NONE',  ( 0.000000000000000000, 0.000000000000000000, 1.000000000000000000 ) ) ;
#83124=CARTESIAN_POINT ( 'NONE',  ( 222.4306832106270804, -141.7221692137691775, 21.50000000000000000 ) ) ;
#83153=CYLINDRICAL_SURFACE ( 'NONE', #24828, 155.4364916446740210 ) ;
#83166=VERTEX_POINT ( 'NONE', #41581 ) ;
#83193=ORIENTED_EDGE ( 'NONE', *, *, #43122, .F. ) ;
#83198=CARTESIAN_POINT ( 'NONE',  ( 222.4306832106270804, -142.7221692137691775, -32.50000000000000711 ) ) ;
#83200=ADVANCED_FACE ( 'NONE', ( #6092 ), #62559, .T. ) ;
#83230=CARTESIAN_POINT ( 'NONE',  ( 123.4306832106270946, -134.2391364535880882, -5.024999999999987921 ) ) ;
#83231=LINE ( 'NONE', #76147, #80600 ) ;
#83250=CONICAL_SURFACE ( 'NONE', #25799, 4.999999999999990230, 1.029744258676648538 ) ;
#83331=CARTESIAN_POINT ( 'NONE',  ( -55.80257052418232888, -229.5268262511776527, -22.50000000000000000 ) ) ;
#83369=DIRECTION ( 'NONE',  ( 0.000000000000000000, -1.000000000000000000, 0.000000000000000000 ) ) ;
#83373=DIRECTION ( 'NONE',  ( 0.000000000000000000, -1.000000000000000000, 0.000000000000000000 ) ) ;
#83377=AXIS2_PLACEMENT_3D ( 'NONE', #83124, #32495, #10693 ) ;
#83410=ORIENTED_EDGE ( 'NONE', *, *, #15163, .T. ) ;
#83427=EDGE_CURVE ( 'NONE', #70176, #5433, #32334, .T. ) ;
#83436=ORIENTED_EDGE ( 'NONE', *, *, #70625, .F. ) ;
#83449=FACE_OUTER_BOUND ( 'NONE', #65204, .T. ) ;
#83467=ORIENTED_EDGE ( 'NONE', *, *, #33278, .F. ) ;
#83482=ORIENTED_EDGE ( 'NONE', *, *, #59045, .T. ) ;
#83506=VECTOR ( 'NONE', #46536, 1000.000000000000000 ) ;
#83513=STYLED_ITEM('',(#93731),#27246);
#83633=ORIENTED_EDGE ( 'NONE', *, *, #74867, .F. ) ;
#83644=AXIS2_PLACEMENT_3D ( 'NONE', #3329, #81010, #10427 ) ;
#83649=VERTEX_POINT ( 'NONE', #15990 ) ;
#83655=AXIS2_PLACEMENT_3D ( 'NONE', #59750, #9513, #81031 ) ;
#83670=AXIS2_PLACEMENT_3D ( 'NONE', #91736, #18376, #19314 ) ;
#83677=CARTESIAN_POINT ( 'NONE',  ( 2.197429475817664013, -229.5268262511776527, 22.50000000000000000 ) ) ;
#83681=CIRCLE ( 'NONE', #26244, 203.9779373800640485 ) ;
#83683=CARTESIAN_POINT ( 'NONE',  ( 194.5881128153457098, 0.000000000000000000, -47.19625681453479871 ) ) ;
#83714=CARTESIAN_POINT ( 'NONE',  ( -18.20453976106250948, -63.49190233628851132, 22.50000000000000000 ) ) ;
#83723=VECTOR ( 'NONE', #39545, 1000.000000000000000 ) ;
#83730=AXIS2_PLACEMENT_3D ( 'NONE', #18875, #5135, #47731 ) ;
#83735=ORIENTED_EDGE ( 'NONE', *, *, #68908, .F. ) ;
#83736=DIRECTION ( 'NONE',  ( -1.000000000000000000, 0.000000000000000000, 0.000000000000000000 ) ) ;
#83737=TOROIDAL_SURFACE ( 'NONE', #53470, 2.000000000000000000, 1.000000000000000000 ) ;
#83756=VERTEX_POINT ( 'NONE', #59076 ) ;
#83781=AXIS2_PLACEMENT_3D ( 'NONE', #29100, #51785, #16744 ) ;
#83792=AXIS2_PLACEMENT_3D ( 'NONE', #38292, #1389, #67207 ) ;
#83826=LINE ( 'NONE', #84753, #5089 ) ;
#83834=CARTESIAN_POINT ( 'NONE',  ( 208.4306832106271088, 42.44233620800392970, 7.500000000000012434 ) ) ;
#83866=CARTESIAN_POINT ( 'NONE',  ( 222.4306832106270804, -141.7221692137691775, 21.50000000000000000 ) ) ;
#83872=VECTOR ( 'NONE', #47184, 1000.000000000000000 ) ;
#83931=DIRECTION ( 'NONE',  ( 1.000000000000000000, 0.000000000000000000, 0.000000000000000000 ) ) ;
#83942=DIRECTION ( 'NONE',  ( 1.000000000000000000, 0.000000000000000000, 0.000000000000000000 ) ) ;
#83970=FACE_OUTER_BOUND ( 'NONE', #47429, .T. ) ;
#84002=ORIENTED_EDGE ( 'NONE', *, *, #1573, .F. ) ;
#84005=ORIENTED_EDGE ( 'NONE', *, *, #16017, .T. ) ;
#84098=CARTESIAN_POINT ( 'NONE',  ( -22.78264641048746597, -118.9815703160634541, 22.50000000000000000 ) ) ;
#84201=CARTESIAN_POINT ( 'NONE',  ( 2.197429475817664013, -229.5268262511776527, -22.50000000000000000 ) ) ;
#84213=ORIENTED_EDGE ( 'NONE', *, *, #74984, .T. ) ;
#84217=DIRECTION ( 'NONE',  ( 0.000000000000000000, 0.000000000000000000, 1.000000000000000000 ) ) ;
#84236=ORIENTED_EDGE ( 'NONE', *, *, #85093, .T. ) ;
#84296=CARTESIAN_POINT ( 'NONE',  ( 194.7510731661265595, -163.7219104664116287, -22.50000000000000000 ) ) ;
#84310=DIRECTION ( 'NONE',  ( -0.000000000000000000, -0.000000000000000000, -1.000000000000000000 ) ) ;
#84323=PLANE ( 'NONE',  #11241 ) ;
#84338=ORIENTED_EDGE ( 'NONE', *, *, #20108, .T. ) ;
#84374=ADVANCED_FACE ( 'NONE', ( #82697 ), #83153, .T. ) ;
#84388=CARTESIAN_POINT ( 'NONE',  ( 194.7510731661265595, -164.3527196417747689, -21.50000000000000000 ) ) ;
#84410=FACE_OUTER_BOUND ( 'NONE', #91720, .T. ) ;
#84459=EDGE_LOOP ( 'NONE', ( #62764, #22864, #92652, #67029 ) ) ;
#84489=EDGE_CURVE ( 'NONE', #74347, #75846, #64210, .T. ) ;
#84529=AXIS2_PLACEMENT_3D ( 'NONE', #19558, #41309, #25263 ) ;
#84539=CARTESIAN_POINT ( 'NONE',  ( 222.4306832106270804, -135.2391364535880882, -22.50000000000000000 ) ) ;
#84608=CARTESIAN_POINT ( 'NONE',  ( 194.5881128153457098, -26.00396092263537540, -47.19625681453479871 ) ) ;
#84664=DIRECTION ( 'NONE',  ( -0.000000000000000000, -0.000000000000000000, -1.000000000000000000 ) ) ;
#84685=ORIENTED_EDGE ( 'NONE', *, *, #68972, .T. ) ;
#84693=DIRECTION ( 'NONE',  ( -0.000000000000000000, -0.000000000000000000, 1.000000000000000000 ) ) ;
#84728=ORIENTED_EDGE ( 'NONE', *, *, #65538, .F. ) ;
#84734=VECTOR ( 'NONE', #71909, 1000.000000000000000 ) ;
#84753=CARTESIAN_POINT ( 'NONE',  ( 169.2744399300530347, -11.64849832608277325, 10.00000000000000000 ) ) ;
#84764=CARTESIAN_POINT ( 'NONE',  ( 222.4306832106270804, -135.2391364535880882, 21.50000000000000000 ) ) ;
#84781=EDGE_CURVE ( 'NONE', #68679, #81769, #18821, .T. ) ;
#84806=ORIENTED_EDGE ( 'NONE', *, *, #11577, .T. ) ;
#84829=ORIENTED_EDGE ( 'NONE', *, *, #80305, .F. ) ;
#84837=CARTESIAN_POINT ( 'NONE',  ( 139.6925840978351516, -141.7221692137691775, 22.50000000000000000 ) ) ;
#84876=CYLINDRICAL_SURFACE ( 'NONE', #37627, 1.000000000000000888 ) ;
#84895=EDGE_LOOP ( 'NONE', ( #58941, #70976, #34962, #45795 ) ) ;
#84897=EDGE_CURVE ( 'NONE', #22426, #77986, #15775, .T. ) ;
#84910=EDGE_CURVE ( 'NONE', #2619, #26019, #81523, .T. ) ;
#84968=APPLICATION_CONTEXT ( 'automotive_design' ) ;
#85075=CARTESIAN_POINT ( 'NONE',  ( 184.7149167944524493, -12.49482340714361506, 10.00000000000000000 ) ) ;
#85093=EDGE_CURVE ( 'NONE', #56465, #41591, #33679, .T. ) ;
#85106=CARTESIAN_POINT ( 'NONE',  ( 61.37083282337847123, -250.8548725835408391, 22.50000000000000000 ) ) ;
#85147=AXIS2_PLACEMENT_3D ( 'NONE', #82296, #1363, #89374 ) ;
#85164=DIRECTION ( 'NONE',  ( -0.000000000000000000, -0.000000000000000000, -1.000000000000000000 ) ) ;
#85180=ORIENTED_EDGE ( 'NONE', *, *, #23115, .F. ) ;
#85239=DIRECTION ( 'NONE',  ( 0.000000000000000000, 0.000000000000000000, -1.000000000000000000 ) ) ;
#85297=VECTOR ( 'NONE', #21195, 1000.000000000000000 ) ;
#85299=AXIS2_PLACEMENT_3D ( 'NONE', #21379, #63100, #49329 ) ;
#85313=CARTESIAN_POINT ( 'NONE',  ( 196.7510731661265595, -141.7221692137691775, -22.50000000000000000 ) ) ;
#85409=CARTESIAN_POINT ( 'NONE',  ( 165.2494399300530290, -11.64849832608277325, 10.00000000000000000 ) ) ;
#85489=DIRECTION ( 'NONE',  ( 0.000000000000000000, 1.000000000000000000, 0.000000000000000000 ) ) ;
#85518=CIRCLE ( 'NONE', #35651, 1.000000000000000888 ) ;
#85533=ORIENTED_EDGE ( 'NONE', *, *, #2712, .F. ) ;
#85548=CARTESIAN_POINT ( 'NONE',  ( 222.8344101925596306, -44.55766379199612004, -21.50000000000000000 ) ) ;
#85549=ADVANCED_FACE ( 'NONE', ( #56418 ), #84323, .F. ) ;
#85555=DIRECTION ( 'NONE',  ( -1.000000000000000000, 0.000000000000000000, 0.000000000000000000 ) ) ;
#85563=ADVANCED_FACE ( 'NONE', ( #90936 ), #18533, .T. ) ;
#85600=PLANE ( 'NONE',  #19999 ) ;
#85679=EDGE_CURVE ( 'NONE', #48629, #6151, #17263, .T. ) ;
#85739=CARTESIAN_POINT ( 'NONE',  ( 236.4625231464875128, -138.0407542764614846, 22.50000000000000000 ) ) ;
#85761=VERTEX_POINT ( 'NONE', #72942 ) ;
#85779=ORIENTED_EDGE ( 'NONE', *, *, #43643, .F. ) ;
#85813=CARTESIAN_POINT ( 'NONE',  ( 60.30156426812553860, -249.1647034777049612, -22.50000000000000000 ) ) ;
#85860=ADVANCED_FACE ( 'NONE', ( #78654 ), #28926, .T. ) ;
#85914=EDGE_CURVE ( 'NONE', #15111, #90289, #91381, .T. ) ;
#85984=DIRECTION ( 'NONE',  ( -1.000000000000000000, 0.000000000000000000, 0.000000000000000000 ) ) ;
#86010=DIRECTION ( 'NONE',  ( -0.000000000000000000, -0.000000000000000000, 1.000000000000000000 ) ) ;
#86056=DIRECTION ( 'NONE',  ( -0.8043439146810398288, 0.5941640067486249066, 0.000000000000000000 ) ) ;
#86060=CARTESIAN_POINT ( 'NONE',  ( -5.802570524182329770, -229.5268262511776527, 22.50000000000000000 ) ) ;
#86071=ORIENTED_EDGE ( 'NONE', *, *, #38265, .F. ) ;
#86091=ORIENTED_EDGE ( 'NONE', *, *, #70625, .T. ) ;
#86098=DIRECTION ( 'NONE',  ( -1.000000000000000000, 8.666672153582269122E-16, 0.000000000000000000 ) ) ;
#86100=CIRCLE ( 'NONE', #15076, 1.000000000000000888 ) ;
#86109=EDGE_LOOP ( 'NONE', ( #45445, #69432, #79147, #38355 ) ) ;
#86150=DIRECTION ( 'NONE',  ( 1.000000000000000000, 0.000000000000000000, -0.000000000000000000 ) ) ;
#86160=AXIS2_PLACEMENT_3D ( 'NONE', #19926, #34611, #32 ) ;
#86161=LINE ( 'NONE', #944, #35435 ) ;
#86165=AXIS2_PLACEMENT_3D ( 'NONE', #80685, #73133, #89167 ) ;
#86185=PLANE ( 'NONE',  #86160 ) ;
#86199=DIRECTION ( 'NONE',  ( 1.000000000000000000, 0.000000000000000000, 0.000000000000000000 ) ) ;
#86200=EDGE_CURVE ( 'NONE', #92063, #43035, #15182, .T. ) ;
#86213=ORIENTED_EDGE ( 'NONE', *, *, #6688, .T. ) ;
#86220=VECTOR ( 'NONE', #51025, 1000.000000000000000 ) ;
#86222=EDGE_LOOP ( 'NONE', ( #23080, #52889 ) ) ;
#86250=DIRECTION ( 'NONE',  ( 0.000000000000000000, 0.000000000000000000, -1.000000000000000000 ) ) ;
#86294=DIRECTION ( 'NONE',  ( -1.000000000000000000, 0.000000000000000000, 0.000000000000000000 ) ) ;
#86325=EDGE_CURVE ( 'NONE', #32648, #7995, #9448, .T. ) ;
#86357=ORIENTED_EDGE ( 'NONE', *, *, #19791, .T. ) ;
#86456=CARTESIAN_POINT ( 'NONE',  ( 222.8344101925596306, -0.9999999999999997780, -22.50000000000000000 ) ) ;
#86457=DIRECTION ( 'NONE',  ( -0.000000000000000000, -0.000000000000000000, 1.000000000000000000 ) ) ;
#86466=DIRECTION ( 'NONE',  ( 0.000000000000000000, -1.000000000000000000, 0.000000000000000000 ) ) ;
#86468=DIRECTION ( 'NONE',  ( -0.000000000000000000, -0.000000000000000000, 1.000000000000000000 ) ) ;
#86470=ORIENTED_EDGE ( 'NONE', *, *, #21629, .F. ) ;
#86544=DIRECTION ( 'NONE',  ( -1.000000000000000000, 0.000000000000000000, 0.000000000000000000 ) ) ;
#86555=AXIS2_PLACEMENT_3D ( 'NONE', #67098, #53813, #76054 ) ;
#86557=DIRECTION ( 'NONE',  ( -0.000000000000000000, -0.000000000000000000, 1.000000000000000000 ) ) ;
#86634=CIRCLE ( 'NONE', #45803, 15.36528803885689420 ) ;
#86648=ORIENTED_EDGE ( 'NONE', *, *, #89784, .T. ) ;
#86680=AXIS2_PLACEMENT_3D ( 'NONE', #60436, #30606, #80798 ) ;
#86759=CIRCLE ( 'NONE', #23230, 0.9999999999999954481 ) ;
#86780=DIRECTION ( 'NONE',  ( -0.000000000000000000, -0.000000000000000000, -1.000000000000000000 ) ) ;
#86802=ORIENTED_EDGE ( 'NONE', *, *, #29222, .T. ) ;
#86831=EDGE_CURVE ( 'NONE', #26085, #50388, #70271, .T. ) ;
#86850=AXIS2_PLACEMENT_3D ( 'NONE', #70195, #35601, #78683 ) ;
#86857=VECTOR ( 'NONE', #81338, 1000.000000000000000 ) ;
#86861=DIRECTION ( 'NONE',  ( -0.000000000000000000, 1.000000000000000000, -0.000000000000000000 ) ) ;
#86864=CONICAL_SURFACE ( 'NONE', #67285, 4.025000000000000355, 0.7853981633973095011 ) ;
#86916=EDGE_CURVE ( 'NONE', #4348, #30831, #23207, .T. ) ;
#86951=ORIENTED_EDGE ( 'NONE', *, *, #73573, .T. ) ;
#87005=CARTESIAN_POINT ( 'NONE',  ( 195.2846006655043141, -165.1985023605670335, 22.50000000000000000 ) ) ;
#87029=DIRECTION ( 'NONE',  ( 0.000000000000000000, 0.000000000000000000, 1.000000000000000000 ) ) ;
#87095=CARTESIAN_POINT ( 'NONE',  ( 222.4306832106270804, -147.4436952405746979, -21.50000000000000000 ) ) ;
#87117=VERTEX_POINT ( 'NONE', #5177 ) ;
#87125=CIRCLE ( 'NONE', #68962, 1.000000000000000888 ) ;
#87153=EDGE_CURVE ( 'NONE', #28617, #56465, #77829, .T. ) ;
#87216=EDGE_CURVE ( 'NONE', #6380, #51697, #4227, .T. ) ;
#87220=ORIENTED_EDGE ( 'NONE', *, *, #17969, .T. ) ;
#87285=EDGE_CURVE ( 'NONE', #93421, #44526, #49096, .T. ) ;
#87287=EDGE_LOOP ( 'NONE', ( #70638, #4592, #27685, #89484 ) ) ;
#87299=CARTESIAN_POINT ( 'NONE',  ( -23.68628624284178130, -55.96374926131388605, 22.50000000000000000 ) ) ;
#87315=DIRECTION ( 'NONE',  ( -0.000000000000000000, -0.000000000000000000, -1.000000000000000000 ) ) ;
#87370=ADVANCED_FACE ( 'NONE', ( #78543 ), #61204, .F. ) ;
#87392=CARTESIAN_POINT ( 'NONE',  ( 195.2846006655043709, -165.1985023605670335, 21.50000000000000000 ) ) ;
#87457=DIRECTION ( 'NONE',  ( 1.000000000000000000, 0.000000000000000000, -0.000000000000000000 ) ) ;
#87492=EDGE_CURVE ( 'NONE', #90289, #15111, #15843, .T. ) ;
#87501=EDGE_CURVE ( 'NONE', #6151, #30132, #34897, .T. ) ;
#87505=FACE_OUTER_BOUND ( 'NONE', #65302, .T. ) ;
#87515=( BOUNDED_CURVE ( )  B_SPLINE_CURVE ( 3, ( #20415, #34, #27509, #72472 ),
 .UNSPECIFIED., .F., .F. ) 
 B_SPLINE_CURVE_WITH_KNOTS ( ( 4, 4 ),
 ( 1.570796326794896558, 3.141592653589793116 ),
 .UNSPECIFIED. ) 
 CURVE ( )  GEOMETRIC_REPRESENTATION_ITEM ( )  RATIONAL_B_SPLINE_CURVE ( ( 1.000000000000000000, 0.8047378541243649375, 0.8047378541243649375, 1.000000000000000000 ) ) 
 REPRESENTATION_ITEM ( '' )  );
#87584=EDGE_LOOP ( 'NONE', ( #12192, #61868, #69, #55502 ) ) ;
#87608=EDGE_LOOP ( 'NONE', ( #68798, #39989, #63937, #1589 ) ) ;
#87626=EDGE_CURVE ( 'NONE', #2619, #51697, #91707, .T. ) ;
#87629=ORIENTED_EDGE ( 'NONE', *, *, #58308, .F. ) ;
#87661=ADVANCED_FACE ( 'NONE', ( #33969 ), #86864, .F. ) ;
#87681=CYLINDRICAL_SURFACE ( 'NONE', #29162, 1.000000000000000888 ) ;
#87696=CIRCLE ( 'NONE', #3092, 155.4364916446740210 ) ;
#87746=VERTEX_POINT ( 'NONE', #42926 ) ;
#87845=EDGE_CURVE ( 'NONE', #30132, #78431, #7084, .T. ) ;
#87857=CARTESIAN_POINT ( 'NONE',  ( -23.40286736638519471, -122.5496321078137356, -21.50000000000000000 ) ) ;
#87863=EDGE_LOOP ( 'NONE', ( #193, #48275, #27327 ) ) ;
#87885=CARTESIAN_POINT ( 'NONE',  ( -5.802570524182329770, -229.5268262511776527, -22.50000000000000000 ) ) ;
#87975=CIRCLE ( 'NONE', #47085, 1.000000000000000888 ) ;
#88004=CARTESIAN_POINT ( 'NONE',  ( 139.6925840978351516, 0.000000000000000000, -21.49999999999998579 ) ) ;
#88011=CARTESIAN_POINT ( 'NONE',  ( -36.09237171215955442, -122.5496321078137356, -22.50000000000000000 ) ) ;
#88027=ADVANCED_FACE ( 'NONE', ( #76671 ), #44610, .F. ) ;
#88037=CARTESIAN_POINT ( 'NONE',  ( 2.197429475817664013, -229.5268262511776527, 22.50000000000000000 ) ) ;
#88055=DIRECTION ( 'NONE',  ( 0.000000000000000000, 0.000000000000000000, -1.000000000000000000 ) ) ;
#88109=AXIS2_PLACEMENT_3D ( 'NONE', #56709, #76596, #85555 ) ;
#88118=DIRECTION ( 'NONE',  ( -0.000000000000000000, -1.000000000000000000, -0.000000000000000000 ) ) ;
#88142=ADVANCED_BREP_SHAPE_REPRESENTATION ( '', ( #27246, #18940 ), #770 ) ;
#88215=ORIENTED_EDGE ( 'NONE', *, *, #53722, .T. ) ;
#88230=DIRECTION ( 'NONE',  ( -0.000000000000000000, 1.000000000000000000, -0.000000000000000000 ) ) ;
#88235=DIRECTION ( 'NONE',  ( -0.000000000000000000, 1.000000000000000000, -0.000000000000000000 ) ) ;
#88261=AXIS2_PLACEMENT_3D ( 'NONE', #35347, #34876, #63788 ) ;
#88311=CIRCLE ( 'NONE', #44452, 4.999999999999990230 ) ;
#88358=CARTESIAN_POINT ( 'NONE',  ( 184.7149167944524493, -12.49482340714361506, 10.00000000000000000 ) ) ;
#88373=DIRECTION ( 'NONE',  ( -0.000000000000000000, 1.000000000000000000, -0.000000000000000000 ) ) ;
#88395=EDGE_CURVE ( 'NONE', #60489, #40992, #32540, .T. ) ;
#88397=VECTOR ( 'NONE', #3317, 1000.000000000000000 ) ;
#88401=ORIENTED_EDGE ( 'NONE', *, *, #70292, .F. ) ;
#88420=ADVANCED_FACE ( 'NONE', ( #42543 ), #6117, .T. ) ;
#88431=EDGE_LOOP ( 'NONE', ( #55139, #24737, #5053, #27342 ) ) ;
#88450=CARTESIAN_POINT ( 'NONE',  ( -36.09237171215955442, -122.5496321078137356, -22.50000000000000000 ) ) ;
#88462=EDGE_LOOP ( 'NONE', ( #57058, #53131, #78752, #41365 ) ) ;
#88481=AXIS2_PLACEMENT_3D ( 'NONE', #28365, #86557, #26950 ) ;
#88570=ORIENTED_EDGE ( 'NONE', *, *, #16793, .T. ) ;
#88592=FACE_OUTER_BOUND ( 'NONE', #36050, .T. ) ;
#88712=DIRECTION ( 'NONE',  ( -1.000000000000000000, 0.000000000000000000, 0.000000000000000000 ) ) ;
#88796=ADVANCED_FACE ( 'NONE', ( #79494 ), #27910, .T. ) ;
#88800=CARTESIAN_POINT ( 'NONE',  ( 60.30377782462291947, -249.1633071459562245, 21.50000000000000000 ) ) ;
#88814=DIRECTION ( 'NONE',  ( 1.000000000000000000, 0.000000000000000000, 0.000000000000000000 ) ) ;
#88855=ORIENTED_EDGE ( 'NONE', *, *, #29222, .F. ) ;
#88867=EDGE_LOOP ( 'NONE', ( #81868, #37216, #46734, #21267 ) ) ;
#88877=DIRECTION ( 'NONE',  ( -0.000000000000000000, -0.000000000000000000, 1.000000000000000000 ) ) ;
#88878=CARTESIAN_POINT ( 'NONE',  ( 194.5881128153457098, -26.00396092263537540, 10.00000000000000178 ) ) ;
#88986=AXIS2_PLACEMENT_3D ( 'NONE', #73138, #8264, #79770 ) ;
#88988=CARTESIAN_POINT ( 'NONE',  ( -23.40286736638519471, -135.2391364535880882, 21.50000000000000000 ) ) ;
#89011=LINE ( 'NONE', #61113, #88397 ) ;
#89045=AXIS2_PLACEMENT_3D ( 'NONE', #45614, #82077, #75002 ) ;
#89112=AXIS2_PLACEMENT_3D ( 'NONE', #59296, #15742, #44602 ) ;
#89116=ORIENTED_EDGE ( 'NONE', *, *, #66220, .T. ) ;
#89167=DIRECTION ( 'NONE',  ( 1.000000000000000000, 0.000000000000000000, 0.000000000000000000 ) ) ;
#89182=CIRCLE ( 'NONE', #7564, 1.000000000000000888 ) ;
#89190=LINE ( 'NONE', #86060, #82103 ) ;
#89239=ORIENTED_EDGE ( 'NONE', *, *, #37291, .F. ) ;
#89247=AXIS2_PLACEMENT_3D ( 'NONE', #44381, #58616, #87457 ) ;
#89281=DIRECTION ( 'NONE',  ( -0.000000000000000000, -0.000000000000000000, -1.000000000000000000 ) ) ;
#89299=FACE_OUTER_BOUND ( 'NONE', #61232, .T. ) ;
#89337=LINE ( 'NONE', #52902, #72030 ) ;
#89372=EDGE_LOOP ( 'NONE', ( #5455, #44062, #72870, #30662 ) ) ;
#89374=DIRECTION ( 'NONE',  ( 0.000000000000000000, 0.000000000000000000, -1.000000000000000000 ) ) ;
#89386=CIRCLE ( 'NONE', #7767, 16.36528803885689598 ) ;
#89403=CARTESIAN_POINT ( 'NONE',  ( 194.7510731661265595, -164.3527196417747405, 21.50000000000000000 ) ) ;
#89415=CARTESIAN_POINT ( 'NONE',  ( 17.06571399127465583, -89.54582641780471874, -22.50000000000000000 ) ) ;
#89484=ORIENTED_EDGE ( 'NONE', *, *, #79409, .T. ) ;
#89485=CYLINDRICAL_SURFACE ( 'NONE', #6564, 1.000000000000000888 ) ;
#89507=AXIS2_PLACEMENT_3D ( 'NONE', #31981, #67043, #3569 ) ;
#89533=DIRECTION ( 'NONE',  ( 0.000000000000000000, 0.000000000000000000, -1.000000000000000000 ) ) ;
#89536=DIRECTION ( 'NONE',  ( 0.000000000000000000, 0.000000000000000000, 1.000000000000000000 ) ) ;
#89540=EDGE_CURVE ( 'NONE', #23241, #60845, #53393, .T. ) ;
#89567=VERTEX_POINT ( 'NONE', #47201 ) ;
#89584=LINE ( 'NONE', #17655, #5231 ) ;
#89625=CARTESIAN_POINT ( 'NONE',  ( -39.80257052418234309, -229.5268262511776527, 22.50000000000000000 ) ) ;
#89652=VECTOR ( 'NONE', #29483, 1000.000000000000000 ) ;
#89674=DIRECTION ( 'NONE',  ( 0.000000000000000000, 0.000000000000000000, 1.000000000000000000 ) ) ;
#89688=ORIENTED_EDGE ( 'NONE', *, *, #73573, .F. ) ;
#89711=ORIENTED_EDGE ( 'NONE', *, *, #92477, .T. ) ;
#89721=PLANE ( 'NONE',  #89507 ) ;
#89731=ADVANCED_FACE ( 'NONE', ( #25446 ), #54323, .T. ) ;
#89784=EDGE_CURVE ( 'NONE', #58890, #73033, #17887, .T. ) ;
#89806=AXIS2_PLACEMENT_3D ( 'NONE', #35535, #58254, #64449 ) ;
#89808=VECTOR ( 'NONE', #22075, 1000.000000000000114 ) ;
#89831=ORIENTED_EDGE ( 'NONE', *, *, #86831, .F. ) ;
#89876=DIRECTION ( 'NONE',  ( -1.000000000000000000, 0.000000000000000000, 0.000000000000000000 ) ) ;
#89879=AXIS2_PLACEMENT_3D ( 'NONE', #3910, #90971, #69238 ) ;
#89891=VECTOR ( 'NONE', #24599, 1000.000000000000114 ) ;
#89906=DIRECTION ( 'NONE',  ( -1.000000000000000000, 2.653393457432135558E-15, 0.000000000000000000 ) ) ;
#89909=EDGE_CURVE ( 'NONE', #34073, #54318, #48616, .T. ) ;
#89985=DIRECTION ( 'NONE',  ( -1.000000000000000000, 0.000000000000000000, 0.000000000000000000 ) ) ;
#90007=ORIENTED_EDGE ( 'NONE', *, *, #14648, .F. ) ;
#90108=VERTEX_POINT ( 'NONE', #70438 ) ;
#90146=EDGE_CURVE ( 'NONE', #79714, #26085, #85518, .T. ) ;
#90187=VERTEX_POINT ( 'NONE', #28728 ) ;
#90219=CARTESIAN_POINT ( 'NONE',  ( 73.43068321062709458, -134.2391364535880598, 4.999999999999990230 ) ) ;
#90249=EDGE_CURVE ( 'NONE', #30132, #19742, #41510, .T. ) ;
#90289=VERTEX_POINT ( 'NONE', #23483 ) ;
#90305=CARTESIAN_POINT ( 'NONE',  ( 222.8344101925596306, -44.55766379199612004, -21.49999999999998579 ) ) ;
#90336=CARTESIAN_POINT ( 'NONE',  ( 125.0516381006429043, 8.053287430127898716, 21.50000000000000000 ) ) ;
#90396=AXIS2_PLACEMENT_3D ( 'NONE', #11438, #90937, #33211 ) ;
#90412=VERTEX_POINT ( 'NONE', #87392 ) ;
#90433=DIRECTION ( 'NONE',  ( 0.000000000000000000, 1.000000000000000000, 0.000000000000000000 ) ) ;
#90500=ORIENTED_EDGE ( 'NONE', *, *, #29763, .F. ) ;
#90518=VERTEX_POINT ( 'NONE', #58085 ) ;
#90569=ORIENTED_EDGE ( 'NONE', *, *, #40534, .T. ) ;
#90632=EDGE_CURVE ( 'NONE', #77294, #4433, #2171, .T. ) ;
#90641=EDGE_CURVE ( 'NONE', #87746, #5433, #52258, .T. ) ;
#90651=AXIS2_PLACEMENT_3D ( 'NONE', #62453, #3270, #10366 ) ;
#90657=AXIS2_PLACEMENT_3D ( 'NONE', #68351, #38977, #61271 ) ;
#90669=LINE ( 'NONE', #90219, #83723 ) ;
#90749=DIRECTION ( 'NONE',  ( 0.000000000000000000, -1.000000000000000000, 0.000000000000000000 ) ) ;
#90766=EDGE_CURVE ( 'NONE', #90187, #44672, #73220, .T. ) ;
#90794=DIRECTION ( 'NONE',  ( -0.000000000000000000, -0.000000000000000000, -1.000000000000000000 ) ) ;
#90812=DIRECTION ( 'NONE',  ( 0.000000000000000000, -1.000000000000000000, 0.000000000000000000 ) ) ;
#90893=EDGE_CURVE ( 'NONE', #59355, #83166, #50780, .T. ) ;
#90936=FACE_OUTER_BOUND ( 'NONE', #48140, .T. ) ;
#90937=DIRECTION ( 'NONE',  ( -1.000000000000000000, 0.000000000000000000, 0.000000000000000000 ) ) ;
#90959=CARTESIAN_POINT ( 'NONE',  ( 0.000000000000000000, 0.000000000000000000, 0.000000000000000000 ) ) ;
#90971=DIRECTION ( 'NONE',  ( -0.000000000000000000, 1.000000000000000000, -0.000000000000000000 ) ) ;
#91037=DIRECTION ( 'NONE',  ( 0.000000000000000000, -1.000000000000000000, 0.000000000000000000 ) ) ;
#91064=MECHANICAL_DESIGN_GEOMETRIC_PRESENTATION_REPRESENTATION('',(#83513),#62396);
#91075=ORIENTED_EDGE ( 'NONE', *, *, #38515, .F. ) ;
#91078=ORIENTED_EDGE ( 'NONE', *, *, #90766, .F. ) ;
#91130=AXIS2_PLACEMENT_3D ( 'NONE', #4847, #76360, #3923 ) ;
#91159=CARTESIAN_POINT ( 'NONE',  ( -23.68628624284178130, -44.55766379199612004, 22.50000000000000000 ) ) ;
#91227=DIRECTION ( 'NONE',  ( 0.000000000000000000, -1.000000000000000000, 0.000000000000000000 ) ) ;
#91232=VECTOR ( 'NONE', #17370, 1000.000000000000000 ) ;
#91272=LINE ( 'NONE', #55329, #25940 ) ;
#91290=AXIS2_PLACEMENT_3D ( 'NONE', #2342, #73380, #74770 ) ;
#91315=ADVANCED_FACE ( 'NONE', ( #71455 ), #77967, .F. ) ;
#91381=CIRCLE ( 'NONE', #43015, 4.025000000000000355 ) ;
#91414=EDGE_LOOP ( 'NONE', ( #28351, #61989, #55267, #52806 ) ) ;
#91431=DIRECTION ( 'NONE',  ( 0.000000000000000000, 0.000000000000000000, -1.000000000000000000 ) ) ;
#91451=ORIENTED_EDGE ( 'NONE', *, *, #37177, .F. ) ;
#91511=FACE_OUTER_BOUND ( 'NONE', #58221, .T. ) ;
#91570=ORIENTED_EDGE ( 'NONE', *, *, #70292, .T. ) ;
#91587=ORIENTED_EDGE ( 'NONE', *, *, #4532, .T. ) ;
#91589=AXIS2_PLACEMENT_3D ( 'NONE', #44309, #14983, #50497 ) ;
#91707=LINE ( 'NONE', #20696, #74849 ) ;
#91720=EDGE_LOOP ( 'NONE', ( #47417, #4672, #92622, #3973 ) ) ;
#91736=CARTESIAN_POINT ( 'NONE',  ( 222.4306832106270804, -141.7221692137691775, -21.50000000000000000 ) ) ;
#91737=EDGE_CURVE ( 'NONE', #28617, #32853, #87125, .T. ) ;
#91750=CARTESIAN_POINT ( 'NONE',  ( 180.6899167944524436, -12.49482340714361506, 10.00000000000000000 ) ) ;
#91774=CARTESIAN_POINT ( 'NONE',  ( 123.4306832106270804, -181.2434395487259167, 0.000000000000000000 ) ) ;
#91785=CYLINDRICAL_SURFACE ( 'NONE', #35007, 7.500000000000012434 ) ;
#91809=ORIENTED_EDGE ( 'NONE', *, *, #77701, .T. ) ;
#91818=DIRECTION ( 'NONE',  ( 0.000000000000000000, -1.000000000000000000, 0.000000000000000000 ) ) ;
#91856=FACE_OUTER_BOUND ( 'NONE', #49313, .T. ) ;
#91869=DIRECTION ( 'NONE',  ( -0.000000000000000000, 1.000000000000000000, 0.000000000000000000 ) ) ;
#91894=DIRECTION ( 'NONE',  ( 0.000000000000000000, 0.000000000000000000, 1.000000000000000000 ) ) ;
#92018=FACE_OUTER_BOUND ( 'NONE', #53093, .T. ) ;
#92033=ORIENTED_EDGE ( 'NONE', *, *, #75740, .F. ) ;
#92063=VERTEX_POINT ( 'NONE', #72832 ) ;
#92095=DIRECTION ( 'NONE',  ( -1.000000000000000000, 0.000000000000000000, 0.000000000000000000 ) ) ;
#92170=ORIENTED_EDGE ( 'NONE', *, *, #73959, .T. ) ;
#92172=CARTESIAN_POINT ( 'NONE',  ( 222.4306832106270804, -135.2391364535880882, -21.50000000000000000 ) ) ;
#92173=DIRECTION ( 'NONE',  ( 1.000000000000000000, -0.000000000000000000, 0.000000000000000000 ) ) ;
#92183=CARTESIAN_POINT ( 'NONE',  ( 195.7510731661265595, -164.3527196417747405, -32.50000000000000711 ) ) ;
#92202=FACE_OUTER_BOUND ( 'NONE', #30197, .T. ) ;
#92241=CIRCLE ( 'NONE', #9090, 1.000000000000000888 ) ;
#92251=ORIENTED_EDGE ( 'NONE', *, *, #68560, .T. ) ;
#92305=AXIS2_PLACEMENT_3D ( 'NONE', #32413, #18664, #68866 ) ;
#92308=EDGE_CURVE ( 'NONE', #89567, #71577, #31155, .T. ) ;
#92325=FACE_OUTER_BOUND ( 'NONE', #67726, .T. ) ;
#92336=CARTESIAN_POINT ( 'NONE',  ( 222.8344101925596590, 7.485601368116228304E-15, -22.08578643762689708 ) ) ;
#92338=CARTESIAN_POINT ( 'NONE',  ( -186.9122233887894140, -89.54582641780471874, 22.50000000000000000 ) ) ;
#92372=AXIS2_PLACEMENT_3D ( 'NONE', #37867, #44970, #67708 ) ;
#92389=ORIENTED_EDGE ( 'NONE', *, *, #40510, .T. ) ;
#92396=DIRECTION ( 'NONE',  ( -1.000000000000000000, 0.000000000000000000, 0.000000000000000000 ) ) ;
#92460=ORIENTED_EDGE ( 'NONE', *, *, #68768, .F. ) ;
#92477=EDGE_CURVE ( 'NONE', #58726, #75846, #89337, .T. ) ;
#92499=ORIENTED_EDGE ( 'NONE', *, *, #42244, .F. ) ;
#92521=VECTOR ( 'NONE', #51453, 1000.000000000000114 ) ;
#92567=CIRCLE ( 'NONE', #63899, 12.40608546931776957 ) ;
#92574=DIRECTION ( 'NONE',  ( -0.000000000000000000, -0.000000000000000000, -1.000000000000000000 ) ) ;
#92592=EDGE_CURVE ( 'NONE', #20083, #87746, #76096, .T. ) ;
#92622=ORIENTED_EDGE ( 'NONE', *, *, #19812, .F. ) ;
#92635=EDGE_LOOP ( 'NONE', ( #20192, #1706, #51946, #44394 ) ) ;
#92640=DIRECTION ( 'NONE',  ( -0.000000000000000000, -0.000000000000000000, -1.000000000000000000 ) ) ;
#92650=VECTOR ( 'NONE', #86010, 1000.000000000000000 ) ;
#92652=ORIENTED_EDGE ( 'NONE', *, *, #64250, .T. ) ;
#92672=VECTOR ( 'NONE', #68259, 1000.000000000000000 ) ;
#92748=VECTOR ( 'NONE', #51144, 1000.000000000000000 ) ;
#92749=EDGE_CURVE ( 'NONE', #93680, #8064, #992, .T. ) ;
#92750=ORIENTED_EDGE ( 'NONE', *, *, #6869, .T. ) ;
#92845=DIRECTION ( 'NONE',  ( 1.000000000000000000, 0.000000000000000000, 0.000000000000000000 ) ) ;
#92955=AXIS2_PLACEMENT_3D ( 'NONE', #10381, #44511, #61078 ) ;
#92963=VECTOR ( 'NONE', #70526, 1000.000000000000000 ) ;
#93020=DIRECTION ( 'NONE',  ( -1.000000000000000000, 0.000000000000000000, 0.000000000000000000 ) ) ;
#93033=LINE ( 'NONE', #27238, #24578 ) ;
#93124=DIRECTION ( 'NONE',  ( -1.000000000000000000, 4.440892098500622123E-13, 0.000000000000000000 ) ) ;
#93161=CARTESIAN_POINT ( 'NONE',  ( 10.41963433625062230, -229.5268262511776527, 21.50000000000000000 ) ) ;
#93211=DIRECTION ( 'NONE',  ( 1.000000000000000000, 0.000000000000000000, 0.000000000000000000 ) ) ;
#93232=CARTESIAN_POINT ( 'NONE',  ( 195.2846006655043425, -165.1985023605670619, -21.50000000000000000 ) ) ;
#93296=ADVANCED_FACE ( 'NONE', ( #13579 ), #46090, .T. ) ;
#93299=EDGE_LOOP ( 'NONE', ( #29534, #53965, #28033, #69603 ) ) ;
#93336=ORIENTED_EDGE ( 'NONE', *, *, #54642, .F. ) ;
#93376=ORIENTED_EDGE ( 'NONE', *, *, #54119, .T. ) ;
#93421=VERTEX_POINT ( 'NONE', #18557 ) ;
#93461=ADVANCED_FACE ( 'NONE', ( #46495 ), #35576, .F. ) ;
#93464=ORIENTED_EDGE ( 'NONE', *, *, #62997, .F. ) ;
#93513=DIRECTION ( 'NONE',  ( -1.224646799147353207E-16, 1.000000000000000000, 0.000000000000000000 ) ) ;
#93570=ORIENTED_EDGE ( 'NONE', *, *, #29763, .T. ) ;
#93583=DIRECTION ( 'NONE',  ( 0.000000000000000000, 0.000000000000000000, 1.000000000000000000 ) ) ;
#93641=ORIENTED_EDGE ( 'NONE', *, *, #8048, .F. ) ;
#93661=ORIENTED_EDGE ( 'NONE', *, *, #20271, .T. ) ;
#93671=AXIS2_PLACEMENT_3D ( 'NONE', #52272, #14910, #16295 ) ;
#93680=VERTEX_POINT ( 'NONE', #53626 ) ;
#93687=ADVANCED_FACE ( 'NONE', ( #46952 ), #3898, .F. ) ;
#93725=COLOUR_RGB('Dark Blue',0.08,0.2,0.34);
#93726=FILL_AREA_STYLE_COLOUR('',#93725);
#93727=FILL_AREA_STYLE('',(#93726));
#93728=SURFACE_STYLE_FILL_AREA(#93727);
#93729=SURFACE_SIDE_STYLE('',(#93728));
#93730=SURFACE_STYLE_USAGE(.BOTH.,#93729);
#93731=PRESENTATION_STYLE_ASSIGNMENT((#93730));
ENDSEC;
END-ISO-10303-21;
